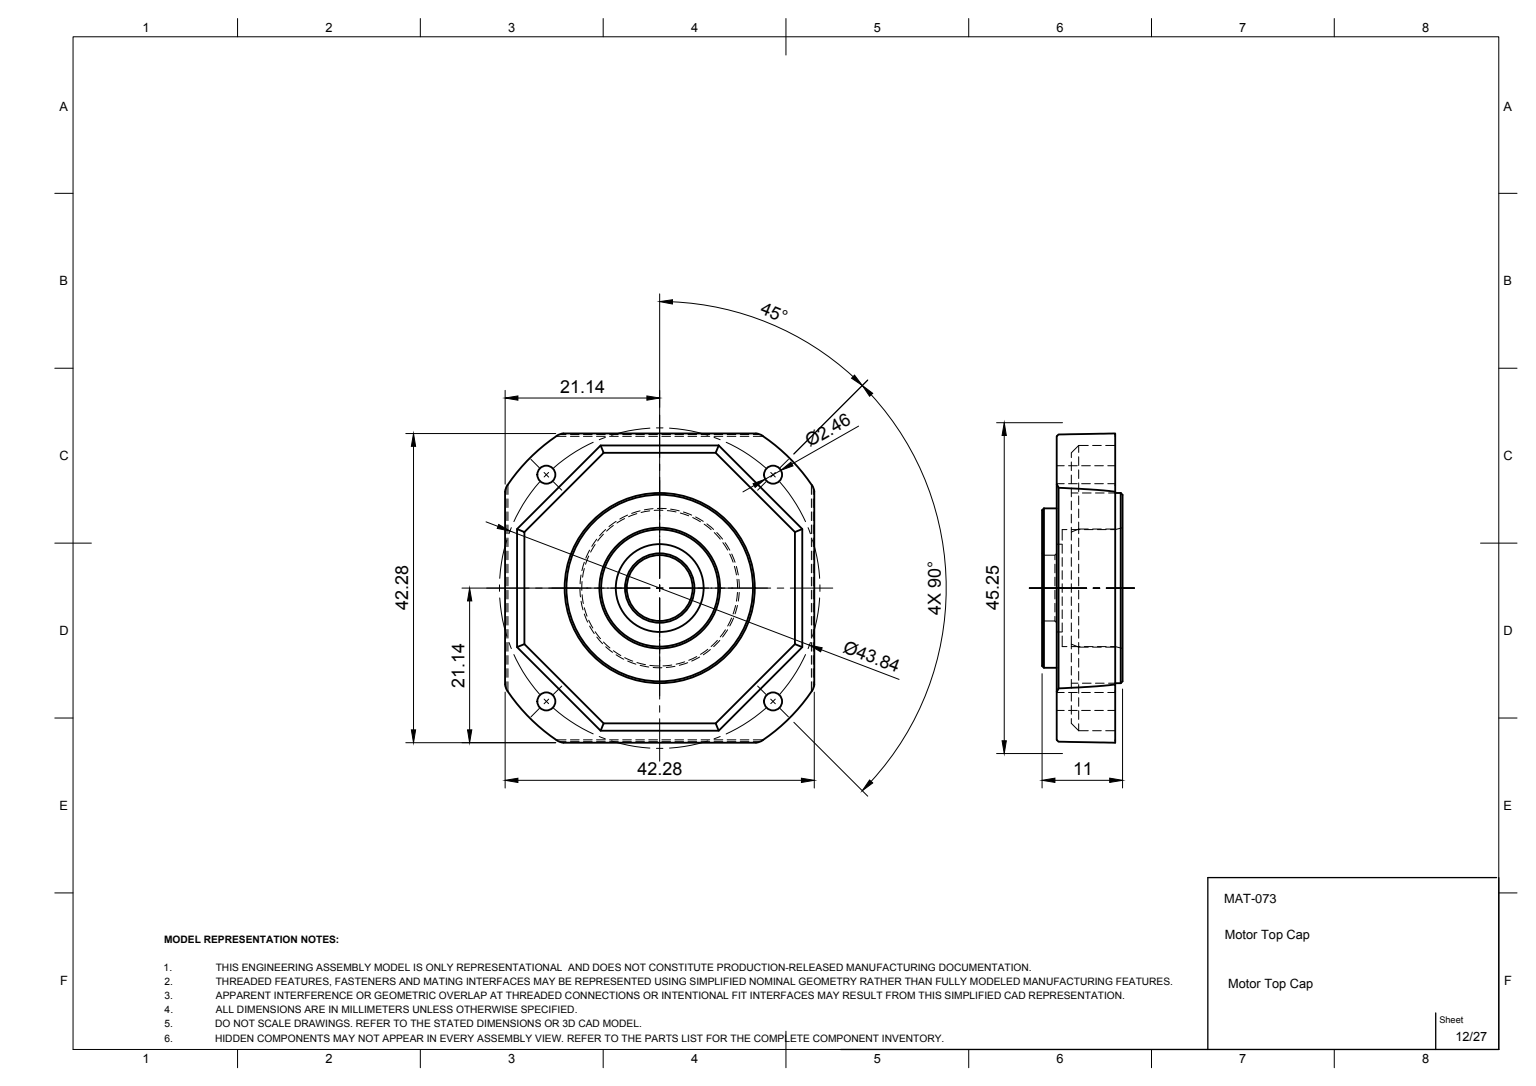
ISO-10303-21;
HEADER;
/* Generated by software containing ST-Developer
 * from STEP Tools, Inc. (www.steptools.com) 
 */

FILE_DESCRIPTION(
/* description */ ('CAx-IF Rec.Pracs.---Representation and Presentation of Product Manufa
cturing Information (PMI)---4.0---2014-10-13'),
/* implementation_level */ '2;1');

FILE_NAME(
/* name */ 'Motor Top Cap.step',
/* time_stamp */ '2026-10-24T18:52:33-07:00',
/* author */ (''),
/* organization */ (''),
/* preprocessor_version */ 'ST-DEVELOPER v20.2',
/* originating_system */ 'Autodesk Translation Framework v15.17.0.0',
/* authorisation */ '');

FILE_SCHEMA (('AP242_MANAGED_MODEL_BASED_3D_ENGINEERING_MIM_LF { 1 0 10303 442 2 1 4 }'));
ENDSEC;

DATA;
#10=MECHANICAL_DESIGN_GEOMETRIC_PRESENTATION_REPRESENTATION('',(#425),#34876);
#180=CONICAL_SURFACE('',#21050,0.010775,0.785398163397447);
#181=CONICAL_SURFACE('',#21057,0.004625,0.785398163397445);
#182=CONICAL_SURFACE('',#21062,0.004625,0.785398163397443);
#183=CONICAL_SURFACE('',#21066,0.012875,0.785398163397446);
#184=CONICAL_SURFACE('',#21072,0.008125,0.244978663126864);
#324=ELLIPSE('',#20968,0.00280406412975229,0.00200000000000295);
#325=ELLIPSE('',#20969,0.114597376997271,0.00200000000000295);
#326=ELLIPSE('',#20972,0.0352260556300016,0.0251250000000291);
#327=ELLIPSE('',#20974,0.0352260556300019,0.0251250000000291);
#328=ELLIPSE('',#20977,0.00280406412976774,0.00200000000001397);
#329=ELLIPSE('',#20978,0.114597376997902,0.00200000000001397);
#330=ELLIPSE('',#20981,0.0352260556299788,0.0251250000000126);
#331=ELLIPSE('',#20983,0.0352260556299788,0.0251250000000126);
#332=ELLIPSE('',#20986,0.00280406412974482,0.00199999999999762);
#333=ELLIPSE('',#20987,0.114597376996966,0.00199999999999762);
#334=ELLIPSE('',#20990,0.0352260556299805,0.0251250000000138);
#335=ELLIPSE('',#20992,0.0352260556299805,0.0251250000000138);
#336=ELLIPSE('',#20995,0.00280406412972858,0.00199999999998605);
#337=ELLIPSE('',#20996,0.114597376996303,0.00199999999998605);
#338=ELLIPSE('',#20999,0.0352260556299806,0.0251250000000138);
#339=ELLIPSE('',#21001,0.0352260556299803,0.0251250000000138);
#340=ELLIPSE('',#21004,0.114597376996528,0.00199999999998998);
#341=ELLIPSE('',#21005,0.00280406412973409,0.00199999999998998);
#342=ELLIPSE('',#21008,0.114597376996513,0.00199999999998973);
#343=ELLIPSE('',#21009,0.00280406412973375,0.00199999999998973);
#344=ELLIPSE('',#21012,0.114597376996527,0.00199999999998997);
#345=ELLIPSE('',#21013,0.00280406412973409,0.00199999999998997);
#346=ELLIPSE('',#21016,0.114597376997844,0.00200000000001296);
#347=ELLIPSE('',#21017,0.00280406412976633,0.00200000000001296);
#359=SHAPE_REPRESENTATION_RELATIONSHIP('SRR','None',#34996,#392);
#392=ADVANCED_BREP_SHAPE_REPRESENTATION('',(#458),#34854);
#425=STYLED_ITEM('',(#35162),#458);
#458=MANIFOLD_SOLID_BREP('Motor Top Cap',#19565);
#519=FACE_BOUND('',#6354,.T.);
#520=FACE_BOUND('',#6355,.T.);
#521=FACE_BOUND('',#6356,.T.);
#522=FACE_BOUND('',#6357,.T.);
#523=FACE_BOUND('',#6358,.T.);
#524=FACE_BOUND('',#6361,.T.);
#525=FACE_BOUND('',#6362,.T.);
#526=FACE_BOUND('',#6363,.T.);
#527=FACE_BOUND('',#6364,.T.);
#528=FACE_BOUND('',#6365,.T.);
#529=FACE_BOUND('',#6379,.T.);
#530=FACE_BOUND('',#6383,.T.);
#531=FACE_BOUND('',#6389,.T.);
#532=FACE_BOUND('',#6392,.T.);
#533=FACE_BOUND('',#6402,.T.);
#816=PLANE('',#21018);
#817=PLANE('',#21019);
#818=PLANE('',#21020);
#819=PLANE('',#21021);
#820=PLANE('',#21022);
#821=PLANE('',#21023);
#822=PLANE('',#21028);
#823=PLANE('',#21029);
#824=PLANE('',#21035);
#825=PLANE('',#21036);
#826=PLANE('',#21037);
#827=PLANE('',#21038);
#828=PLANE('',#21039);
#829=PLANE('',#21040);
#830=PLANE('',#21041);
#831=PLANE('',#21042);
#832=PLANE('',#21043);
#833=PLANE('',#21044);
#834=PLANE('',#21045);
#835=PLANE('',#21046);
#836=PLANE('',#21047);
#837=PLANE('',#21049);
#838=PLANE('',#21054);
#839=PLANE('',#21064);
#840=PLANE('',#21069);
#841=PLANE('',#21083);
#842=PLANE('',#21084);
#843=PLANE('',#21085);
#844=PLANE('',#21086);
#845=PLANE('',#21087);
#846=PLANE('',#21088);
#1767=LINE('',#31314,#3366);
#1768=LINE('',#31322,#3367);
#1769=LINE('',#31333,#3368);
#1770=LINE('',#31341,#3369);
#1771=LINE('',#31352,#3370);
#1772=LINE('',#31360,#3371);
#1773=LINE('',#31371,#3372);
#1774=LINE('',#31379,#3373);
#1775=LINE('',#31410,#3374);
#1776=LINE('',#31411,#3375);
#1777=LINE('',#31413,#3376);
#1778=LINE('',#31415,#3377);
#1779=LINE('',#31416,#3378);
#1780=LINE('',#31418,#3379);
#1781=LINE('',#31420,#3380);
#1782=LINE('',#31421,#3381);
#1783=LINE('',#31423,#3382);
#1784=LINE('',#31426,#3383);
#1785=LINE('',#31428,#3384);
#1786=LINE('',#31430,#3385);
#1787=LINE('',#31432,#3386);
#1788=LINE('',#31434,#3387);
#1789=LINE('',#31436,#3388);
#1790=LINE('',#31438,#3389);
#1791=LINE('',#31439,#3390);
#1792=LINE('',#31449,#3391);
#1793=LINE('',#31451,#3392);
#1794=LINE('',#31465,#3393);
#1795=LINE('',#31467,#3394);
#1796=LINE('',#31469,#3395);
#1797=LINE('',#31470,#3396);
#1798=LINE('',#31473,#3397);
#1799=LINE('',#31475,#3398);
#1800=LINE('',#31476,#3399);
#1801=LINE('',#31479,#3400);
#1802=LINE('',#31481,#3401);
#1803=LINE('',#31482,#3402);
#1804=LINE('',#31485,#3403);
#1805=LINE('',#31487,#3404);
#1806=LINE('',#31488,#3405);
#1807=LINE('',#31491,#3406);
#1808=LINE('',#31493,#3407);
#1809=LINE('',#31494,#3408);
#1810=LINE('',#31497,#3409);
#1811=LINE('',#31499,#3410);
#1812=LINE('',#31500,#3411);
#1813=LINE('',#31503,#3412);
#1814=LINE('',#31505,#3413);
#1815=LINE('',#31506,#3414);
#1816=LINE('',#31508,#3415);
#1817=LINE('',#31509,#3416);
#1818=LINE('',#31511,#3417);
#1819=LINE('',#31512,#3418);
#1820=LINE('',#31514,#3419);
#1821=LINE('',#31516,#3420);
#1822=LINE('',#31518,#3421);
#1823=LINE('',#31523,#3422);
#1824=LINE('',#31529,#3423);
#1825=LINE('',#31536,#3424);
#1826=LINE('',#31541,#3425);
#1827=LINE('',#31546,#3426);
#1828=LINE('',#31549,#3427);
#1829=LINE('',#31558,#3428);
#1830=LINE('',#31564,#3429);
#1831=LINE('',#31569,#3430);
#1832=LINE('',#31573,#3431);
#1833=LINE('',#31576,#3432);
#1834=LINE('',#31578,#3433);
#1835=LINE('',#31580,#3434);
#1836=LINE('',#31582,#3435);
#1837=LINE('',#31586,#3436);
#1838=LINE('',#31589,#3437);
#1839=LINE('',#31591,#3438);
#1840=LINE('',#31593,#3439);
#3366=VECTOR('',#24976,0.01);
#3367=VECTOR('',#24985,0.01);
#3368=VECTOR('',#24996,0.01);
#3369=VECTOR('',#25005,0.01);
#3370=VECTOR('',#25016,0.01);
#3371=VECTOR('',#25025,0.01);
#3372=VECTOR('',#25036,0.01);
#3373=VECTOR('',#25045,0.01);
#3374=VECTOR('',#25086,1.);
#3375=VECTOR('',#25087,1.);
#3376=VECTOR('',#25090,1.);
#3377=VECTOR('',#25093,1.);
#3378=VECTOR('',#25094,1.);
#3379=VECTOR('',#25097,1.);
#3380=VECTOR('',#25100,1.);
#3381=VECTOR('',#25101,1.);
#3382=VECTOR('',#25104,1.);
#3383=VECTOR('',#25105,1.);
#3384=VECTOR('',#25106,1.);
#3385=VECTOR('',#25107,1.);
#3386=VECTOR('',#25108,1.);
#3387=VECTOR('',#25109,1.);
#3388=VECTOR('',#25110,1.);
#3389=VECTOR('',#25111,1.);
#3390=VECTOR('',#25112,1.);
#3391=VECTOR('',#25123,1.);
#3392=VECTOR('',#25126,1.);
#3393=VECTOR('',#25139,1.);
#3394=VECTOR('',#25140,1.);
#3395=VECTOR('',#25141,1.);
#3396=VECTOR('',#25142,1.);
#3397=VECTOR('',#25145,1.);
#3398=VECTOR('',#25146,1.);
#3399=VECTOR('',#25147,1.);
#3400=VECTOR('',#25150,1.);
#3401=VECTOR('',#25151,1.);
#3402=VECTOR('',#25152,1.);
#3403=VECTOR('',#25155,1.);
#3404=VECTOR('',#25156,1.);
#3405=VECTOR('',#25157,1.);
#3406=VECTOR('',#25160,1.);
#3407=VECTOR('',#25161,1.);
#3408=VECTOR('',#25162,1.);
#3409=VECTOR('',#25165,1.);
#3410=VECTOR('',#25166,1.);
#3411=VECTOR('',#25167,1.);
#3412=VECTOR('',#25170,1.);
#3413=VECTOR('',#25171,1.);
#3414=VECTOR('',#25172,1.);
#3415=VECTOR('',#25175,1.);
#3416=VECTOR('',#25176,1.);
#3417=VECTOR('',#25179,1.);
#3418=VECTOR('',#25180,1.);
#3419=VECTOR('',#25183,1.);
#3420=VECTOR('',#25186,1.);
#3421=VECTOR('',#25189,1.);
#3422=VECTOR('',#25196,1.);
#3423=VECTOR('',#25201,0.010775);
#3424=VECTOR('',#25212,0.0109);
#3425=VECTOR('',#25217,0.004625);
#3426=VECTOR('',#25224,0.0045);
#3427=VECTOR('',#25227,0.004625);
#3428=VECTOR('',#25238,0.012875);
#3429=VECTOR('',#25247,0.013);
#3430=VECTOR('',#25252,0.008125);
#3431=VECTOR('',#25257,0.008);
#3432=VECTOR('',#25262,0.0012295);
#3433=VECTOR('',#25265,0.0012295);
#3434=VECTOR('',#25268,0.0012295);
#3435=VECTOR('',#25271,0.0012295);
#3436=VECTOR('',#25276,0.006);
#3437=VECTOR('',#25281,1.);
#3438=VECTOR('',#25284,1.);
#3439=VECTOR('',#25287,1.);
#4504=CYLINDRICAL_SURFACE('',#20966,0.00200000000000295);
#4505=CYLINDRICAL_SURFACE('',#20970,0.0251250000000291);
#4506=CYLINDRICAL_SURFACE('',#20975,0.00200000000001397);
#4507=CYLINDRICAL_SURFACE('',#20979,0.0251250000000126);
#4508=CYLINDRICAL_SURFACE('',#20984,0.00199999999999762);
#4509=CYLINDRICAL_SURFACE('',#20988,0.0251250000000138);
#4510=CYLINDRICAL_SURFACE('',#20993,0.00199999999998605);
#4511=CYLINDRICAL_SURFACE('',#20997,0.0251250000000138);
#4512=CYLINDRICAL_SURFACE('',#21002,0.00199999999998998);
#4513=CYLINDRICAL_SURFACE('',#21006,0.00199999999998973);
#4514=CYLINDRICAL_SURFACE('',#21010,0.00199999999998997);
#4515=CYLINDRICAL_SURFACE('',#21014,0.00200000000001296);
#4516=CYLINDRICAL_SURFACE('',#21056,0.0109);
#4517=CYLINDRICAL_SURFACE('',#21060,0.0045);
#4518=CYLINDRICAL_SURFACE('',#21071,0.013);
#4519=CYLINDRICAL_SURFACE('',#21075,0.008);
#4520=CYLINDRICAL_SURFACE('',#21077,0.0012295);
#4521=CYLINDRICAL_SURFACE('',#21078,0.0012295);
#4522=CYLINDRICAL_SURFACE('',#21079,0.0012295);
#4523=CYLINDRICAL_SURFACE('',#21080,0.0012295);
#4524=CYLINDRICAL_SURFACE('',#21081,0.006);
#5252=FACE_OUTER_BOUND('',#6336,.T.);
#5253=FACE_OUTER_BOUND('',#6337,.T.);
#5254=FACE_OUTER_BOUND('',#6338,.T.);
#5255=FACE_OUTER_BOUND('',#6339,.T.);
#5256=FACE_OUTER_BOUND('',#6340,.T.);
#5257=FACE_OUTER_BOUND('',#6341,.T.);
#5258=FACE_OUTER_BOUND('',#6342,.T.);
#5259=FACE_OUTER_BOUND('',#6343,.T.);
#5260=FACE_OUTER_BOUND('',#6344,.T.);
#5261=FACE_OUTER_BOUND('',#6345,.T.);
#5262=FACE_OUTER_BOUND('',#6346,.T.);
#5263=FACE_OUTER_BOUND('',#6347,.T.);
#5264=FACE_OUTER_BOUND('',#6348,.T.);
#5265=FACE_OUTER_BOUND('',#6349,.T.);
#5266=FACE_OUTER_BOUND('',#6350,.T.);
#5267=FACE_OUTER_BOUND('',#6351,.T.);
#5268=FACE_OUTER_BOUND('',#6352,.T.);
#5269=FACE_OUTER_BOUND('',#6353,.T.);
#5270=FACE_OUTER_BOUND('',#6359,.T.);
#5271=FACE_OUTER_BOUND('',#6360,.T.);
#5272=FACE_OUTER_BOUND('',#6366,.T.);
#5273=FACE_OUTER_BOUND('',#6367,.T.);
#5274=FACE_OUTER_BOUND('',#6368,.T.);
#5275=FACE_OUTER_BOUND('',#6369,.T.);
#5276=FACE_OUTER_BOUND('',#6370,.T.);
#5277=FACE_OUTER_BOUND('',#6371,.T.);
#5278=FACE_OUTER_BOUND('',#6372,.T.);
#5279=FACE_OUTER_BOUND('',#6373,.T.);
#5280=FACE_OUTER_BOUND('',#6374,.T.);
#5281=FACE_OUTER_BOUND('',#6375,.T.);
#5282=FACE_OUTER_BOUND('',#6376,.T.);
#5283=FACE_OUTER_BOUND('',#6377,.T.);
#5284=FACE_OUTER_BOUND('',#6378,.T.);
#5285=FACE_OUTER_BOUND('',#6380,.T.);
#5286=FACE_OUTER_BOUND('',#6381,.T.);
#5287=FACE_OUTER_BOUND('',#6382,.T.);
#5288=FACE_OUTER_BOUND('',#6384,.T.);
#5289=FACE_OUTER_BOUND('',#6385,.T.);
#5290=FACE_OUTER_BOUND('',#6386,.T.);
#5291=FACE_OUTER_BOUND('',#6387,.T.);
#5292=FACE_OUTER_BOUND('',#6388,.T.);
#5293=FACE_OUTER_BOUND('',#6390,.T.);
#5294=FACE_OUTER_BOUND('',#6391,.T.);
#5295=FACE_OUTER_BOUND('',#6393,.T.);
#5296=FACE_OUTER_BOUND('',#6394,.T.);
#5297=FACE_OUTER_BOUND('',#6395,.T.);
#5298=FACE_OUTER_BOUND('',#6396,.T.);
#5299=FACE_OUTER_BOUND('',#6397,.T.);
#5300=FACE_OUTER_BOUND('',#6398,.T.);
#5301=FACE_OUTER_BOUND('',#6399,.T.);
#5302=FACE_OUTER_BOUND('',#6400,.T.);
#5303=FACE_OUTER_BOUND('',#6401,.T.);
#5304=FACE_OUTER_BOUND('',#6403,.T.);
#5305=FACE_OUTER_BOUND('',#6404,.T.);
#5306=FACE_OUTER_BOUND('',#6405,.T.);
#5307=FACE_OUTER_BOUND('',#6406,.T.);
#5308=FACE_OUTER_BOUND('',#6407,.T.);
#6336=EDGE_LOOP('',(#15300,#15301,#15302,#15303));
#6337=EDGE_LOOP('',(#15304,#15305,#15306,#15307,#15308,#15309));
#6338=EDGE_LOOP('',(#15310,#15311,#15312,#15313));
#6339=EDGE_LOOP('',(#15314,#15315,#15316,#15317,#15318,#15319));
#6340=EDGE_LOOP('',(#15320,#15321,#15322,#15323));
#6341=EDGE_LOOP('',(#15324,#15325,#15326,#15327,#15328,#15329));
#6342=EDGE_LOOP('',(#15330,#15331,#15332,#15333));
#6343=EDGE_LOOP('',(#15334,#15335,#15336,#15337,#15338,#15339));
#6344=EDGE_LOOP('',(#15340,#15341,#15342,#15343));
#6345=EDGE_LOOP('',(#15344,#15345,#15346,#15347));
#6346=EDGE_LOOP('',(#15348,#15349,#15350,#15351));
#6347=EDGE_LOOP('',(#15352,#15353,#15354,#15355));
#6348=EDGE_LOOP('',(#15356,#15357,#15358,#15359));
#6349=EDGE_LOOP('',(#15360,#15361,#15362,#15363,#15364,#15365));
#6350=EDGE_LOOP('',(#15366,#15367,#15368,#15369));
#6351=EDGE_LOOP('',(#15370,#15371,#15372,#15373,#15374,#15375));
#6352=EDGE_LOOP('',(#15376,#15377,#15378,#15379));
#6353=EDGE_LOOP('',(#15380,#15381,#15382,#15383,#15384,#15385,#15386,#15387,
#15388,#15389,#15390,#15391,#15392,#15393,#15394,#15395));
#6354=EDGE_LOOP('',(#15396,#15397,#15398,#15399,#15400,#15401,#15402,#15403));
#6355=EDGE_LOOP('',(#15404));
#6356=EDGE_LOOP('',(#15405));
#6357=EDGE_LOOP('',(#15406));
#6358=EDGE_LOOP('',(#15407));
#6359=EDGE_LOOP('',(#15408,#15409,#15410,#15411,#15412,#15413));
#6360=EDGE_LOOP('',(#15414,#15415,#15416,#15417,#15418,#15419,#15420,#15421));
#6361=EDGE_LOOP('',(#15422));
#6362=EDGE_LOOP('',(#15423));
#6363=EDGE_LOOP('',(#15424));
#6364=EDGE_LOOP('',(#15425));
#6365=EDGE_LOOP('',(#15426));
#6366=EDGE_LOOP('',(#15427,#15428,#15429,#15430));
#6367=EDGE_LOOP('',(#15431,#15432,#15433,#15434));
#6368=EDGE_LOOP('',(#15435,#15436,#15437,#15438));
#6369=EDGE_LOOP('',(#15439,#15440,#15441,#15442));
#6370=EDGE_LOOP('',(#15443,#15444,#15445,#15446));
#6371=EDGE_LOOP('',(#15447,#15448,#15449,#15450));
#6372=EDGE_LOOP('',(#15451,#15452,#15453,#15454));
#6373=EDGE_LOOP('',(#15455,#15456,#15457,#15458));
#6374=EDGE_LOOP('',(#15459,#15460,#15461,#15462));
#6375=EDGE_LOOP('',(#15463,#15464,#15465,#15466));
#6376=EDGE_LOOP('',(#15467,#15468,#15469,#15470));
#6377=EDGE_LOOP('',(#15471,#15472,#15473,#15474));
#6378=EDGE_LOOP('',(#15475,#15476,#15477,#15478,#15479,#15480,#15481,#15482));
#6379=EDGE_LOOP('',(#15483));
#6380=EDGE_LOOP('',(#15484,#15485,#15486,#15487,#15488,#15489));
#6381=EDGE_LOOP('',(#15490,#15491,#15492,#15493,#15494));
#6382=EDGE_LOOP('',(#15495));
#6383=EDGE_LOOP('',(#15496));
#6384=EDGE_LOOP('',(#15497,#15498,#15499,#15500,#15501));
#6385=EDGE_LOOP('',(#15502,#15503,#15504,#15505,#15506));
#6386=EDGE_LOOP('',(#15507,#15508,#15509,#15510,#15511));
#6387=EDGE_LOOP('',(#15512,#15513,#15514,#15515));
#6388=EDGE_LOOP('',(#15516));
#6389=EDGE_LOOP('',(#15517));
#6390=EDGE_LOOP('',(#15518,#15519,#15520,#15521));
#6391=EDGE_LOOP('',(#15522));
#6392=EDGE_LOOP('',(#15523));
#6393=EDGE_LOOP('',(#15524,#15525,#15526,#15527));
#6394=EDGE_LOOP('',(#15528,#15529,#15530,#15531,#15532));
#6395=EDGE_LOOP('',(#15533,#15534,#15535,#15536,#15537));
#6396=EDGE_LOOP('',(#15538,#15539,#15540,#15541));
#6397=EDGE_LOOP('',(#15542,#15543,#15544,#15545));
#6398=EDGE_LOOP('',(#15546,#15547,#15548,#15549));
#6399=EDGE_LOOP('',(#15550,#15551,#15552,#15553));
#6400=EDGE_LOOP('',(#15554,#15555,#15556,#15557));
#6401=EDGE_LOOP('',(#15558));
#6402=EDGE_LOOP('',(#15559));
#6403=EDGE_LOOP('',(#15560,#15561,#15562,#15563));
#6404=EDGE_LOOP('',(#15564,#15565,#15566,#15567));
#6405=EDGE_LOOP('',(#15568,#15569,#15570,#15571));
#6406=EDGE_LOOP('',(#15572,#15573,#15574,#15575));
#6407=EDGE_LOOP('',(#15576,#15577,#15578,#15579));
#7448=CIRCLE('',#20967,0.00200000000000295);
#7449=CIRCLE('',#20971,0.0251250000000291);
#7450=CIRCLE('',#20973,0.0251250000000291);
#7451=CIRCLE('',#20976,0.00200000000001397);
#7452=CIRCLE('',#20980,0.0251250000000126);
#7453=CIRCLE('',#20982,0.0251250000000126);
#7454=CIRCLE('',#20985,0.00199999999999762);
#7455=CIRCLE('',#20989,0.0251250000000138);
#7456=CIRCLE('',#20991,0.0251250000000138);
#7457=CIRCLE('',#20994,0.00199999999998605);
#7458=CIRCLE('',#20998,0.0251250000000138);
#7459=CIRCLE('',#21000,0.0251250000000138);
#7460=CIRCLE('',#21003,0.00199999999998998);
#7461=CIRCLE('',#21007,0.00199999999998973);
#7462=CIRCLE('',#21011,0.00199999999998997);
#7463=CIRCLE('',#21015,0.00200000000001296);
#7464=CIRCLE('',#21024,0.00122950000001);
#7465=CIRCLE('',#21025,0.00122950000001);
#7466=CIRCLE('',#21026,0.00122950000001);
#7467=CIRCLE('',#21027,0.00122950000001);
#7468=CIRCLE('',#21030,0.00122950000001);
#7469=CIRCLE('',#21031,0.00122950000001);
#7470=CIRCLE('',#21032,0.00122950000001);
#7471=CIRCLE('',#21033,0.00122950000001);
#7472=CIRCLE('',#21034,0.01090000000001);
#7473=CIRCLE('',#21048,0.01300000000001);
#7474=CIRCLE('',#21051,0.01090000000001);
#7475=CIRCLE('',#21052,0.01065000000001);
#7476=CIRCLE('',#21053,0.01090000000001);
#7477=CIRCLE('',#21055,0.00475000000001);
#7478=CIRCLE('',#21058,0.00450000000001);
#7479=CIRCLE('',#21059,0.00450000000001);
#7480=CIRCLE('',#21061,0.00450000000001);
#7481=CIRCLE('',#21063,0.00475000000001);
#7482=CIRCLE('',#21065,0.00600000000001);
#7483=CIRCLE('',#21067,0.01300000000001);
#7484=CIRCLE('',#21068,0.01275000000001);
#7485=CIRCLE('',#21070,0.00825000000001);
#7486=CIRCLE('',#21073,0.00800000000001);
#7487=CIRCLE('',#21074,0.00800000000001);
#7488=CIRCLE('',#21076,0.00800000000001);
#7489=CIRCLE('',#21082,0.00600000000001);
#8900=VERTEX_POINT('',#31310);
#8901=VERTEX_POINT('',#31311);
#8902=VERTEX_POINT('',#31313);
#8903=VERTEX_POINT('',#31315);
#8904=VERTEX_POINT('',#31319);
#8905=VERTEX_POINT('',#31321);
#8906=VERTEX_POINT('',#31323);
#8907=VERTEX_POINT('',#31325);
#8908=VERTEX_POINT('',#31329);
#8909=VERTEX_POINT('',#31330);
#8910=VERTEX_POINT('',#31332);
#8911=VERTEX_POINT('',#31334);
#8912=VERTEX_POINT('',#31338);
#8913=VERTEX_POINT('',#31340);
#8914=VERTEX_POINT('',#31342);
#8915=VERTEX_POINT('',#31344);
#8916=VERTEX_POINT('',#31348);
#8917=VERTEX_POINT('',#31349);
#8918=VERTEX_POINT('',#31351);
#8919=VERTEX_POINT('',#31353);
#8920=VERTEX_POINT('',#31357);
#8921=VERTEX_POINT('',#31359);
#8922=VERTEX_POINT('',#31361);
#8923=VERTEX_POINT('',#31363);
#8924=VERTEX_POINT('',#31367);
#8925=VERTEX_POINT('',#31368);
#8926=VERTEX_POINT('',#31370);
#8927=VERTEX_POINT('',#31372);
#8928=VERTEX_POINT('',#31376);
#8929=VERTEX_POINT('',#31378);
#8930=VERTEX_POINT('',#31380);
#8931=VERTEX_POINT('',#31382);
#8932=VERTEX_POINT('',#31386);
#8933=VERTEX_POINT('',#31388);
#8934=VERTEX_POINT('',#31392);
#8935=VERTEX_POINT('',#31394);
#8936=VERTEX_POINT('',#31398);
#8937=VERTEX_POINT('',#31400);
#8938=VERTEX_POINT('',#31404);
#8939=VERTEX_POINT('',#31406);
#8940=VERTEX_POINT('',#31424);
#8941=VERTEX_POINT('',#31425);
#8942=VERTEX_POINT('',#31427);
#8943=VERTEX_POINT('',#31429);
#8944=VERTEX_POINT('',#31431);
#8945=VERTEX_POINT('',#31433);
#8946=VERTEX_POINT('',#31435);
#8947=VERTEX_POINT('',#31437);
#8948=VERTEX_POINT('',#31440);
#8949=VERTEX_POINT('',#31442);
#8950=VERTEX_POINT('',#31444);
#8951=VERTEX_POINT('',#31446);
#8952=VERTEX_POINT('',#31452);
#8953=VERTEX_POINT('',#31454);
#8954=VERTEX_POINT('',#31456);
#8955=VERTEX_POINT('',#31458);
#8956=VERTEX_POINT('',#31460);
#8957=VERTEX_POINT('',#31463);
#8958=VERTEX_POINT('',#31464);
#8959=VERTEX_POINT('',#31466);
#8960=VERTEX_POINT('',#31468);
#8961=VERTEX_POINT('',#31472);
#8962=VERTEX_POINT('',#31474);
#8963=VERTEX_POINT('',#31478);
#8964=VERTEX_POINT('',#31480);
#8965=VERTEX_POINT('',#31484);
#8966=VERTEX_POINT('',#31486);
#8967=VERTEX_POINT('',#31490);
#8968=VERTEX_POINT('',#31492);
#8969=VERTEX_POINT('',#31496);
#8970=VERTEX_POINT('',#31498);
#8971=VERTEX_POINT('',#31502);
#8972=VERTEX_POINT('',#31504);
#8973=VERTEX_POINT('',#31520);
#8974=VERTEX_POINT('',#31525);
#8975=VERTEX_POINT('',#31526);
#8976=VERTEX_POINT('',#31528);
#8977=VERTEX_POINT('',#31533);
#8978=VERTEX_POINT('',#31538);
#8979=VERTEX_POINT('',#31539);
#8980=VERTEX_POINT('',#31544);
#8981=VERTEX_POINT('',#31548);
#8982=VERTEX_POINT('',#31552);
#8983=VERTEX_POINT('',#31555);
#8984=VERTEX_POINT('',#31557);
#8985=VERTEX_POINT('',#31561);
#8986=VERTEX_POINT('',#31566);
#8987=VERTEX_POINT('',#31567);
#8988=VERTEX_POINT('',#31572);
#8989=VERTEX_POINT('',#31584);
#11208=EDGE_CURVE('',#8900,#8901,#7448,.T.);
#11209=EDGE_CURVE('',#8902,#8900,#1767,.T.);
#11210=EDGE_CURVE('',#8903,#8902,#324,.T.);
#11211=EDGE_CURVE('',#8901,#8903,#325,.T.);
#11212=EDGE_CURVE('',#8904,#8900,#7449,.T.);
#11213=EDGE_CURVE('',#8905,#8904,#1768,.T.);
#11214=EDGE_CURVE('',#8906,#8905,#326,.T.);
#11215=EDGE_CURVE('',#8907,#8906,#7450,.T.);
#11216=EDGE_CURVE('',#8902,#8907,#327,.T.);
#11217=EDGE_CURVE('',#8908,#8909,#7451,.T.);
#11218=EDGE_CURVE('',#8910,#8908,#1769,.T.);
#11219=EDGE_CURVE('',#8911,#8910,#328,.T.);
#11220=EDGE_CURVE('',#8909,#8911,#329,.T.);
#11221=EDGE_CURVE('',#8912,#8908,#7452,.T.);
#11222=EDGE_CURVE('',#8913,#8912,#1770,.T.);
#11223=EDGE_CURVE('',#8914,#8913,#330,.T.);
#11224=EDGE_CURVE('',#8915,#8914,#7453,.T.);
#11225=EDGE_CURVE('',#8910,#8915,#331,.T.);
#11226=EDGE_CURVE('',#8916,#8917,#7454,.T.);
#11227=EDGE_CURVE('',#8918,#8916,#1771,.T.);
#11228=EDGE_CURVE('',#8919,#8918,#332,.T.);
#11229=EDGE_CURVE('',#8917,#8919,#333,.T.);
#11230=EDGE_CURVE('',#8920,#8916,#7455,.T.);
#11231=EDGE_CURVE('',#8921,#8920,#1772,.T.);
#11232=EDGE_CURVE('',#8922,#8921,#334,.T.);
#11233=EDGE_CURVE('',#8923,#8922,#7456,.T.);
#11234=EDGE_CURVE('',#8918,#8923,#335,.T.);
#11235=EDGE_CURVE('',#8924,#8925,#7457,.T.);
#11236=EDGE_CURVE('',#8926,#8924,#1773,.T.);
#11237=EDGE_CURVE('',#8927,#8926,#336,.T.);
#11238=EDGE_CURVE('',#8925,#8927,#337,.T.);
#11239=EDGE_CURVE('',#8928,#8924,#7458,.T.);
#11240=EDGE_CURVE('',#8929,#8928,#1774,.T.);
#11241=EDGE_CURVE('',#8930,#8929,#338,.T.);
#11242=EDGE_CURVE('',#8931,#8930,#7459,.T.);
#11243=EDGE_CURVE('',#8926,#8931,#339,.T.);
#11244=EDGE_CURVE('',#8932,#8904,#7460,.T.);
#11245=EDGE_CURVE('',#8933,#8932,#340,.T.);
#11246=EDGE_CURVE('',#8905,#8933,#341,.T.);
#11247=EDGE_CURVE('',#8934,#8912,#7461,.T.);
#11248=EDGE_CURVE('',#8935,#8934,#342,.T.);
#11249=EDGE_CURVE('',#8913,#8935,#343,.T.);
#11250=EDGE_CURVE('',#8936,#8920,#7462,.T.);
#11251=EDGE_CURVE('',#8937,#8936,#344,.T.);
#11252=EDGE_CURVE('',#8921,#8937,#345,.T.);
#11253=EDGE_CURVE('',#8938,#8928,#7463,.T.);
#11254=EDGE_CURVE('',#8939,#8938,#346,.T.);
#11255=EDGE_CURVE('',#8929,#8939,#347,.T.);
#11256=EDGE_CURVE('',#8935,#8903,#1775,.T.);
#11257=EDGE_CURVE('',#8934,#8901,#1776,.T.);
#11258=EDGE_CURVE('',#8907,#8914,#1777,.T.);
#11259=EDGE_CURVE('',#8937,#8911,#1778,.T.);
#11260=EDGE_CURVE('',#8936,#8909,#1779,.T.);
#11261=EDGE_CURVE('',#8915,#8922,#1780,.T.);
#11262=EDGE_CURVE('',#8939,#8919,#1781,.T.);
#11263=EDGE_CURVE('',#8938,#8917,#1782,.T.);
#11264=EDGE_CURVE('',#8932,#8925,#1783,.T.);
#11265=EDGE_CURVE('',#8940,#8941,#1784,.T.);
#11266=EDGE_CURVE('',#8941,#8942,#1785,.T.);
#11267=EDGE_CURVE('',#8942,#8943,#1786,.T.);
#11268=EDGE_CURVE('',#8943,#8944,#1787,.T.);
#11269=EDGE_CURVE('',#8944,#8945,#1788,.T.);
#11270=EDGE_CURVE('',#8945,#8946,#1789,.T.);
#11271=EDGE_CURVE('',#8946,#8947,#1790,.T.);
#11272=EDGE_CURVE('',#8947,#8940,#1791,.T.);
#11273=EDGE_CURVE('',#8948,#8948,#7464,.T.);
#11274=EDGE_CURVE('',#8949,#8949,#7465,.T.);
#11275=EDGE_CURVE('',#8950,#8950,#7466,.T.);
#11276=EDGE_CURVE('',#8951,#8951,#7467,.T.);
#11277=EDGE_CURVE('',#8923,#8930,#1792,.T.);
#11278=EDGE_CURVE('',#8931,#8906,#1793,.T.);
#11279=EDGE_CURVE('',#8952,#8952,#7468,.T.);
#11280=EDGE_CURVE('',#8953,#8953,#7469,.T.);
#11281=EDGE_CURVE('',#8954,#8954,#7470,.T.);
#11282=EDGE_CURVE('',#8955,#8955,#7471,.T.);
#11283=EDGE_CURVE('',#8956,#8956,#7472,.T.);
#11284=EDGE_CURVE('',#8957,#8958,#1794,.T.);
#11285=EDGE_CURVE('',#8958,#8959,#1795,.T.);
#11286=EDGE_CURVE('',#8959,#8960,#1796,.T.);
#11287=EDGE_CURVE('',#8957,#8960,#1797,.T.);
#11288=EDGE_CURVE('',#8958,#8961,#1798,.T.);
#11289=EDGE_CURVE('',#8961,#8962,#1799,.T.);
#11290=EDGE_CURVE('',#8962,#8959,#1800,.T.);
#11291=EDGE_CURVE('',#8961,#8963,#1801,.T.);
#11292=EDGE_CURVE('',#8963,#8964,#1802,.T.);
#11293=EDGE_CURVE('',#8964,#8962,#1803,.T.);
#11294=EDGE_CURVE('',#8965,#8964,#1804,.T.);
#11295=EDGE_CURVE('',#8963,#8966,#1805,.T.);
#11296=EDGE_CURVE('',#8966,#8965,#1806,.T.);
#11297=EDGE_CURVE('',#8967,#8965,#1807,.T.);
#11298=EDGE_CURVE('',#8966,#8968,#1808,.T.);
#11299=EDGE_CURVE('',#8968,#8967,#1809,.T.);
#11300=EDGE_CURVE('',#8969,#8967,#1810,.T.);
#11301=EDGE_CURVE('',#8968,#8970,#1811,.T.);
#11302=EDGE_CURVE('',#8970,#8969,#1812,.T.);
#11303=EDGE_CURVE('',#8971,#8969,#1813,.T.);
#11304=EDGE_CURVE('',#8970,#8972,#1814,.T.);
#11305=EDGE_CURVE('',#8972,#8971,#1815,.T.);
#11306=EDGE_CURVE('',#8960,#8971,#1816,.T.);
#11307=EDGE_CURVE('',#8972,#8957,#1817,.T.);
#11308=EDGE_CURVE('',#8947,#8969,#1818,.T.);
#11309=EDGE_CURVE('',#8946,#8967,#1819,.T.);
#11310=EDGE_CURVE('',#8940,#8971,#1820,.T.);
#11311=EDGE_CURVE('',#8941,#8960,#1821,.T.);
#11312=EDGE_CURVE('',#8942,#8959,#1822,.T.);
#11313=EDGE_CURVE('',#8973,#8973,#7473,.T.);
#11314=EDGE_CURVE('',#8933,#8927,#1823,.T.);
#11315=EDGE_CURVE('',#8974,#8975,#7474,.T.);
#11316=EDGE_CURVE('',#8975,#8976,#1824,.T.);
#11317=EDGE_CURVE('',#8976,#8976,#7475,.T.);
#11318=EDGE_CURVE('',#8975,#8974,#7476,.T.);
#11319=EDGE_CURVE('',#8977,#8977,#7477,.T.);
#11320=EDGE_CURVE('',#8974,#8956,#1825,.T.);
#11321=EDGE_CURVE('',#8978,#8979,#7478,.T.);
#11322=EDGE_CURVE('',#8979,#8977,#1826,.T.);
#11323=EDGE_CURVE('',#8979,#8978,#7479,.T.);
#11324=EDGE_CURVE('',#8980,#8980,#7480,.T.);
#11325=EDGE_CURVE('',#8980,#8978,#1827,.T.);
#11326=EDGE_CURVE('',#8980,#8981,#1828,.T.);
#11327=EDGE_CURVE('',#8981,#8981,#7481,.T.);
#11328=EDGE_CURVE('',#8982,#8982,#7482,.T.);
#11329=EDGE_CURVE('',#8983,#8983,#7483,.T.);
#11330=EDGE_CURVE('',#8983,#8984,#1829,.T.);
#11331=EDGE_CURVE('',#8984,#8984,#7484,.T.);
#11332=EDGE_CURVE('',#8985,#8985,#7485,.T.);
#11333=EDGE_CURVE('',#8973,#8983,#1830,.T.);
#11334=EDGE_CURVE('',#8986,#8987,#7486,.T.);
#11335=EDGE_CURVE('',#8987,#8985,#1831,.T.);
#11336=EDGE_CURVE('',#8987,#8986,#7487,.T.);
#11337=EDGE_CURVE('',#8986,#8988,#1832,.T.);
#11338=EDGE_CURVE('',#8988,#8988,#7488,.T.);
#11339=EDGE_CURVE('',#8951,#8952,#1833,.T.);
#11340=EDGE_CURVE('',#8950,#8953,#1834,.T.);
#11341=EDGE_CURVE('',#8949,#8954,#1835,.T.);
#11342=EDGE_CURVE('',#8948,#8955,#1836,.T.);
#11343=EDGE_CURVE('',#8989,#8989,#7489,.T.);
#11344=EDGE_CURVE('',#8989,#8982,#1837,.T.);
#11345=EDGE_CURVE('',#8945,#8965,#1838,.T.);
#11346=EDGE_CURVE('',#8944,#8964,#1839,.T.);
#11347=EDGE_CURVE('',#8943,#8962,#1840,.T.);
#15300=ORIENTED_EDGE('',*,*,#11208,.F.);
#15301=ORIENTED_EDGE('',*,*,#11209,.F.);
#15302=ORIENTED_EDGE('',*,*,#11210,.F.);
#15303=ORIENTED_EDGE('',*,*,#11211,.F.);
#15304=ORIENTED_EDGE('',*,*,#11212,.F.);
#15305=ORIENTED_EDGE('',*,*,#11213,.F.);
#15306=ORIENTED_EDGE('',*,*,#11214,.F.);
#15307=ORIENTED_EDGE('',*,*,#11215,.F.);
#15308=ORIENTED_EDGE('',*,*,#11216,.F.);
#15309=ORIENTED_EDGE('',*,*,#11209,.T.);
#15310=ORIENTED_EDGE('',*,*,#11217,.F.);
#15311=ORIENTED_EDGE('',*,*,#11218,.F.);
#15312=ORIENTED_EDGE('',*,*,#11219,.F.);
#15313=ORIENTED_EDGE('',*,*,#11220,.F.);
#15314=ORIENTED_EDGE('',*,*,#11221,.F.);
#15315=ORIENTED_EDGE('',*,*,#11222,.F.);
#15316=ORIENTED_EDGE('',*,*,#11223,.F.);
#15317=ORIENTED_EDGE('',*,*,#11224,.F.);
#15318=ORIENTED_EDGE('',*,*,#11225,.F.);
#15319=ORIENTED_EDGE('',*,*,#11218,.T.);
#15320=ORIENTED_EDGE('',*,*,#11226,.F.);
#15321=ORIENTED_EDGE('',*,*,#11227,.F.);
#15322=ORIENTED_EDGE('',*,*,#11228,.F.);
#15323=ORIENTED_EDGE('',*,*,#11229,.F.);
#15324=ORIENTED_EDGE('',*,*,#11230,.F.);
#15325=ORIENTED_EDGE('',*,*,#11231,.F.);
#15326=ORIENTED_EDGE('',*,*,#11232,.F.);
#15327=ORIENTED_EDGE('',*,*,#11233,.F.);
#15328=ORIENTED_EDGE('',*,*,#11234,.F.);
#15329=ORIENTED_EDGE('',*,*,#11227,.T.);
#15330=ORIENTED_EDGE('',*,*,#11235,.F.);
#15331=ORIENTED_EDGE('',*,*,#11236,.F.);
#15332=ORIENTED_EDGE('',*,*,#11237,.F.);
#15333=ORIENTED_EDGE('',*,*,#11238,.F.);
#15334=ORIENTED_EDGE('',*,*,#11239,.F.);
#15335=ORIENTED_EDGE('',*,*,#11240,.F.);
#15336=ORIENTED_EDGE('',*,*,#11241,.F.);
#15337=ORIENTED_EDGE('',*,*,#11242,.F.);
#15338=ORIENTED_EDGE('',*,*,#11243,.F.);
#15339=ORIENTED_EDGE('',*,*,#11236,.T.);
#15340=ORIENTED_EDGE('',*,*,#11244,.F.);
#15341=ORIENTED_EDGE('',*,*,#11245,.F.);
#15342=ORIENTED_EDGE('',*,*,#11246,.F.);
#15343=ORIENTED_EDGE('',*,*,#11213,.T.);
#15344=ORIENTED_EDGE('',*,*,#11247,.F.);
#15345=ORIENTED_EDGE('',*,*,#11248,.F.);
#15346=ORIENTED_EDGE('',*,*,#11249,.F.);
#15347=ORIENTED_EDGE('',*,*,#11222,.T.);
#15348=ORIENTED_EDGE('',*,*,#11250,.F.);
#15349=ORIENTED_EDGE('',*,*,#11251,.F.);
#15350=ORIENTED_EDGE('',*,*,#11252,.F.);
#15351=ORIENTED_EDGE('',*,*,#11231,.T.);
#15352=ORIENTED_EDGE('',*,*,#11253,.F.);
#15353=ORIENTED_EDGE('',*,*,#11254,.F.);
#15354=ORIENTED_EDGE('',*,*,#11255,.F.);
#15355=ORIENTED_EDGE('',*,*,#11240,.T.);
#15356=ORIENTED_EDGE('',*,*,#11211,.T.);
#15357=ORIENTED_EDGE('',*,*,#11256,.F.);
#15358=ORIENTED_EDGE('',*,*,#11248,.T.);
#15359=ORIENTED_EDGE('',*,*,#11257,.T.);
#15360=ORIENTED_EDGE('',*,*,#11210,.T.);
#15361=ORIENTED_EDGE('',*,*,#11216,.T.);
#15362=ORIENTED_EDGE('',*,*,#11258,.T.);
#15363=ORIENTED_EDGE('',*,*,#11223,.T.);
#15364=ORIENTED_EDGE('',*,*,#11249,.T.);
#15365=ORIENTED_EDGE('',*,*,#11256,.T.);
#15366=ORIENTED_EDGE('',*,*,#11220,.T.);
#15367=ORIENTED_EDGE('',*,*,#11259,.F.);
#15368=ORIENTED_EDGE('',*,*,#11251,.T.);
#15369=ORIENTED_EDGE('',*,*,#11260,.T.);
#15370=ORIENTED_EDGE('',*,*,#11219,.T.);
#15371=ORIENTED_EDGE('',*,*,#11225,.T.);
#15372=ORIENTED_EDGE('',*,*,#11261,.T.);
#15373=ORIENTED_EDGE('',*,*,#11232,.T.);
#15374=ORIENTED_EDGE('',*,*,#11252,.T.);
#15375=ORIENTED_EDGE('',*,*,#11259,.T.);
#15376=ORIENTED_EDGE('',*,*,#11229,.T.);
#15377=ORIENTED_EDGE('',*,*,#11262,.F.);
#15378=ORIENTED_EDGE('',*,*,#11254,.T.);
#15379=ORIENTED_EDGE('',*,*,#11263,.T.);
#15380=ORIENTED_EDGE('',*,*,#11244,.T.);
#15381=ORIENTED_EDGE('',*,*,#11212,.T.);
#15382=ORIENTED_EDGE('',*,*,#11208,.T.);
#15383=ORIENTED_EDGE('',*,*,#11257,.F.);
#15384=ORIENTED_EDGE('',*,*,#11247,.T.);
#15385=ORIENTED_EDGE('',*,*,#11221,.T.);
#15386=ORIENTED_EDGE('',*,*,#11217,.T.);
#15387=ORIENTED_EDGE('',*,*,#11260,.F.);
#15388=ORIENTED_EDGE('',*,*,#11250,.T.);
#15389=ORIENTED_EDGE('',*,*,#11230,.T.);
#15390=ORIENTED_EDGE('',*,*,#11226,.T.);
#15391=ORIENTED_EDGE('',*,*,#11263,.F.);
#15392=ORIENTED_EDGE('',*,*,#11253,.T.);
#15393=ORIENTED_EDGE('',*,*,#11239,.T.);
#15394=ORIENTED_EDGE('',*,*,#11235,.T.);
#15395=ORIENTED_EDGE('',*,*,#11264,.F.);
#15396=ORIENTED_EDGE('',*,*,#11265,.T.);
#15397=ORIENTED_EDGE('',*,*,#11266,.T.);
#15398=ORIENTED_EDGE('',*,*,#11267,.T.);
#15399=ORIENTED_EDGE('',*,*,#11268,.T.);
#15400=ORIENTED_EDGE('',*,*,#11269,.T.);
#15401=ORIENTED_EDGE('',*,*,#11270,.T.);
#15402=ORIENTED_EDGE('',*,*,#11271,.T.);
#15403=ORIENTED_EDGE('',*,*,#11272,.T.);
#15404=ORIENTED_EDGE('',*,*,#11273,.T.);
#15405=ORIENTED_EDGE('',*,*,#11274,.T.);
#15406=ORIENTED_EDGE('',*,*,#11275,.T.);
#15407=ORIENTED_EDGE('',*,*,#11276,.T.);
#15408=ORIENTED_EDGE('',*,*,#11228,.T.);
#15409=ORIENTED_EDGE('',*,*,#11234,.T.);
#15410=ORIENTED_EDGE('',*,*,#11277,.T.);
#15411=ORIENTED_EDGE('',*,*,#11241,.T.);
#15412=ORIENTED_EDGE('',*,*,#11255,.T.);
#15413=ORIENTED_EDGE('',*,*,#11262,.T.);
#15414=ORIENTED_EDGE('',*,*,#11215,.T.);
#15415=ORIENTED_EDGE('',*,*,#11278,.F.);
#15416=ORIENTED_EDGE('',*,*,#11242,.T.);
#15417=ORIENTED_EDGE('',*,*,#11277,.F.);
#15418=ORIENTED_EDGE('',*,*,#11233,.T.);
#15419=ORIENTED_EDGE('',*,*,#11261,.F.);
#15420=ORIENTED_EDGE('',*,*,#11224,.T.);
#15421=ORIENTED_EDGE('',*,*,#11258,.F.);
#15422=ORIENTED_EDGE('',*,*,#11279,.T.);
#15423=ORIENTED_EDGE('',*,*,#11280,.T.);
#15424=ORIENTED_EDGE('',*,*,#11281,.T.);
#15425=ORIENTED_EDGE('',*,*,#11282,.T.);
#15426=ORIENTED_EDGE('',*,*,#11283,.T.);
#15427=ORIENTED_EDGE('',*,*,#11284,.T.);
#15428=ORIENTED_EDGE('',*,*,#11285,.T.);
#15429=ORIENTED_EDGE('',*,*,#11286,.T.);
#15430=ORIENTED_EDGE('',*,*,#11287,.F.);
#15431=ORIENTED_EDGE('',*,*,#11288,.T.);
#15432=ORIENTED_EDGE('',*,*,#11289,.T.);
#15433=ORIENTED_EDGE('',*,*,#11290,.T.);
#15434=ORIENTED_EDGE('',*,*,#11285,.F.);
#15435=ORIENTED_EDGE('',*,*,#11291,.T.);
#15436=ORIENTED_EDGE('',*,*,#11292,.T.);
#15437=ORIENTED_EDGE('',*,*,#11293,.T.);
#15438=ORIENTED_EDGE('',*,*,#11289,.F.);
#15439=ORIENTED_EDGE('',*,*,#11294,.T.);
#15440=ORIENTED_EDGE('',*,*,#11292,.F.);
#15441=ORIENTED_EDGE('',*,*,#11295,.T.);
#15442=ORIENTED_EDGE('',*,*,#11296,.T.);
#15443=ORIENTED_EDGE('',*,*,#11297,.T.);
#15444=ORIENTED_EDGE('',*,*,#11296,.F.);
#15445=ORIENTED_EDGE('',*,*,#11298,.T.);
#15446=ORIENTED_EDGE('',*,*,#11299,.T.);
#15447=ORIENTED_EDGE('',*,*,#11300,.T.);
#15448=ORIENTED_EDGE('',*,*,#11299,.F.);
#15449=ORIENTED_EDGE('',*,*,#11301,.T.);
#15450=ORIENTED_EDGE('',*,*,#11302,.T.);
#15451=ORIENTED_EDGE('',*,*,#11303,.T.);
#15452=ORIENTED_EDGE('',*,*,#11302,.F.);
#15453=ORIENTED_EDGE('',*,*,#11304,.T.);
#15454=ORIENTED_EDGE('',*,*,#11305,.T.);
#15455=ORIENTED_EDGE('',*,*,#11306,.T.);
#15456=ORIENTED_EDGE('',*,*,#11305,.F.);
#15457=ORIENTED_EDGE('',*,*,#11307,.T.);
#15458=ORIENTED_EDGE('',*,*,#11287,.T.);
#15459=ORIENTED_EDGE('',*,*,#11300,.F.);
#15460=ORIENTED_EDGE('',*,*,#11308,.F.);
#15461=ORIENTED_EDGE('',*,*,#11271,.F.);
#15462=ORIENTED_EDGE('',*,*,#11309,.T.);
#15463=ORIENTED_EDGE('',*,*,#11303,.F.);
#15464=ORIENTED_EDGE('',*,*,#11310,.F.);
#15465=ORIENTED_EDGE('',*,*,#11272,.F.);
#15466=ORIENTED_EDGE('',*,*,#11308,.T.);
#15467=ORIENTED_EDGE('',*,*,#11306,.F.);
#15468=ORIENTED_EDGE('',*,*,#11311,.F.);
#15469=ORIENTED_EDGE('',*,*,#11265,.F.);
#15470=ORIENTED_EDGE('',*,*,#11310,.T.);
#15471=ORIENTED_EDGE('',*,*,#11286,.F.);
#15472=ORIENTED_EDGE('',*,*,#11312,.F.);
#15473=ORIENTED_EDGE('',*,*,#11266,.F.);
#15474=ORIENTED_EDGE('',*,*,#11311,.T.);
#15475=ORIENTED_EDGE('',*,*,#11284,.F.);
#15476=ORIENTED_EDGE('',*,*,#11307,.F.);
#15477=ORIENTED_EDGE('',*,*,#11304,.F.);
#15478=ORIENTED_EDGE('',*,*,#11301,.F.);
#15479=ORIENTED_EDGE('',*,*,#11298,.F.);
#15480=ORIENTED_EDGE('',*,*,#11295,.F.);
#15481=ORIENTED_EDGE('',*,*,#11291,.F.);
#15482=ORIENTED_EDGE('',*,*,#11288,.F.);
#15483=ORIENTED_EDGE('',*,*,#11313,.F.);
#15484=ORIENTED_EDGE('',*,*,#11246,.T.);
#15485=ORIENTED_EDGE('',*,*,#11314,.T.);
#15486=ORIENTED_EDGE('',*,*,#11237,.T.);
#15487=ORIENTED_EDGE('',*,*,#11243,.T.);
#15488=ORIENTED_EDGE('',*,*,#11278,.T.);
#15489=ORIENTED_EDGE('',*,*,#11214,.T.);
#15490=ORIENTED_EDGE('',*,*,#11315,.T.);
#15491=ORIENTED_EDGE('',*,*,#11316,.T.);
#15492=ORIENTED_EDGE('',*,*,#11317,.T.);
#15493=ORIENTED_EDGE('',*,*,#11316,.F.);
#15494=ORIENTED_EDGE('',*,*,#11318,.T.);
#15495=ORIENTED_EDGE('',*,*,#11317,.F.);
#15496=ORIENTED_EDGE('',*,*,#11319,.F.);
#15497=ORIENTED_EDGE('',*,*,#11315,.F.);
#15498=ORIENTED_EDGE('',*,*,#11320,.T.);
#15499=ORIENTED_EDGE('',*,*,#11283,.F.);
#15500=ORIENTED_EDGE('',*,*,#11320,.F.);
#15501=ORIENTED_EDGE('',*,*,#11318,.F.);
#15502=ORIENTED_EDGE('',*,*,#11321,.T.);
#15503=ORIENTED_EDGE('',*,*,#11322,.T.);
#15504=ORIENTED_EDGE('',*,*,#11319,.T.);
#15505=ORIENTED_EDGE('',*,*,#11322,.F.);
#15506=ORIENTED_EDGE('',*,*,#11323,.T.);
#15507=ORIENTED_EDGE('',*,*,#11324,.F.);
#15508=ORIENTED_EDGE('',*,*,#11325,.T.);
#15509=ORIENTED_EDGE('',*,*,#11323,.F.);
#15510=ORIENTED_EDGE('',*,*,#11321,.F.);
#15511=ORIENTED_EDGE('',*,*,#11325,.F.);
#15512=ORIENTED_EDGE('',*,*,#11324,.T.);
#15513=ORIENTED_EDGE('',*,*,#11326,.T.);
#15514=ORIENTED_EDGE('',*,*,#11327,.T.);
#15515=ORIENTED_EDGE('',*,*,#11326,.F.);
#15516=ORIENTED_EDGE('',*,*,#11328,.F.);
#15517=ORIENTED_EDGE('',*,*,#11327,.F.);
#15518=ORIENTED_EDGE('',*,*,#11329,.T.);
#15519=ORIENTED_EDGE('',*,*,#11330,.T.);
#15520=ORIENTED_EDGE('',*,*,#11331,.T.);
#15521=ORIENTED_EDGE('',*,*,#11330,.F.);
#15522=ORIENTED_EDGE('',*,*,#11331,.F.);
#15523=ORIENTED_EDGE('',*,*,#11332,.F.);
#15524=ORIENTED_EDGE('',*,*,#11313,.T.);
#15525=ORIENTED_EDGE('',*,*,#11333,.T.);
#15526=ORIENTED_EDGE('',*,*,#11329,.F.);
#15527=ORIENTED_EDGE('',*,*,#11333,.F.);
#15528=ORIENTED_EDGE('',*,*,#11334,.T.);
#15529=ORIENTED_EDGE('',*,*,#11335,.T.);
#15530=ORIENTED_EDGE('',*,*,#11332,.T.);
#15531=ORIENTED_EDGE('',*,*,#11335,.F.);
#15532=ORIENTED_EDGE('',*,*,#11336,.T.);
#15533=ORIENTED_EDGE('',*,*,#11334,.F.);
#15534=ORIENTED_EDGE('',*,*,#11337,.T.);
#15535=ORIENTED_EDGE('',*,*,#11338,.T.);
#15536=ORIENTED_EDGE('',*,*,#11337,.F.);
#15537=ORIENTED_EDGE('',*,*,#11336,.F.);
#15538=ORIENTED_EDGE('',*,*,#11276,.F.);
#15539=ORIENTED_EDGE('',*,*,#11339,.T.);
#15540=ORIENTED_EDGE('',*,*,#11279,.F.);
#15541=ORIENTED_EDGE('',*,*,#11339,.F.);
#15542=ORIENTED_EDGE('',*,*,#11275,.F.);
#15543=ORIENTED_EDGE('',*,*,#11340,.T.);
#15544=ORIENTED_EDGE('',*,*,#11280,.F.);
#15545=ORIENTED_EDGE('',*,*,#11340,.F.);
#15546=ORIENTED_EDGE('',*,*,#11274,.F.);
#15547=ORIENTED_EDGE('',*,*,#11341,.T.);
#15548=ORIENTED_EDGE('',*,*,#11281,.F.);
#15549=ORIENTED_EDGE('',*,*,#11341,.F.);
#15550=ORIENTED_EDGE('',*,*,#11273,.F.);
#15551=ORIENTED_EDGE('',*,*,#11342,.T.);
#15552=ORIENTED_EDGE('',*,*,#11282,.F.);
#15553=ORIENTED_EDGE('',*,*,#11342,.F.);
#15554=ORIENTED_EDGE('',*,*,#11343,.F.);
#15555=ORIENTED_EDGE('',*,*,#11344,.T.);
#15556=ORIENTED_EDGE('',*,*,#11328,.T.);
#15557=ORIENTED_EDGE('',*,*,#11344,.F.);
#15558=ORIENTED_EDGE('',*,*,#11338,.F.);
#15559=ORIENTED_EDGE('',*,*,#11343,.T.);
#15560=ORIENTED_EDGE('',*,*,#11297,.F.);
#15561=ORIENTED_EDGE('',*,*,#11309,.F.);
#15562=ORIENTED_EDGE('',*,*,#11270,.F.);
#15563=ORIENTED_EDGE('',*,*,#11345,.T.);
#15564=ORIENTED_EDGE('',*,*,#11294,.F.);
#15565=ORIENTED_EDGE('',*,*,#11345,.F.);
#15566=ORIENTED_EDGE('',*,*,#11269,.F.);
#15567=ORIENTED_EDGE('',*,*,#11346,.T.);
#15568=ORIENTED_EDGE('',*,*,#11293,.F.);
#15569=ORIENTED_EDGE('',*,*,#11346,.F.);
#15570=ORIENTED_EDGE('',*,*,#11268,.F.);
#15571=ORIENTED_EDGE('',*,*,#11347,.T.);
#15572=ORIENTED_EDGE('',*,*,#11290,.F.);
#15573=ORIENTED_EDGE('',*,*,#11347,.F.);
#15574=ORIENTED_EDGE('',*,*,#11267,.F.);
#15575=ORIENTED_EDGE('',*,*,#11312,.T.);
#15576=ORIENTED_EDGE('',*,*,#11245,.T.);
#15577=ORIENTED_EDGE('',*,*,#11264,.T.);
#15578=ORIENTED_EDGE('',*,*,#11238,.T.);
#15579=ORIENTED_EDGE('',*,*,#11314,.F.);
#18968=ADVANCED_FACE('',(#5252),#4504,.T.);
#18969=ADVANCED_FACE('',(#5253),#4505,.T.);
#18970=ADVANCED_FACE('',(#5254),#4506,.T.);
#18971=ADVANCED_FACE('',(#5255),#4507,.T.);
#18972=ADVANCED_FACE('',(#5256),#4508,.T.);
#18973=ADVANCED_FACE('',(#5257),#4509,.T.);
#18974=ADVANCED_FACE('',(#5258),#4510,.T.);
#18975=ADVANCED_FACE('',(#5259),#4511,.T.);
#18976=ADVANCED_FACE('',(#5260),#4512,.T.);
#18977=ADVANCED_FACE('',(#5261),#4513,.T.);
#18978=ADVANCED_FACE('',(#5262),#4514,.T.);
#18979=ADVANCED_FACE('',(#5263),#4515,.T.);
#18980=ADVANCED_FACE('',(#5264),#816,.T.);
#18981=ADVANCED_FACE('',(#5265),#817,.T.);
#18982=ADVANCED_FACE('',(#5266),#818,.T.);
#18983=ADVANCED_FACE('',(#5267),#819,.T.);
#18984=ADVANCED_FACE('',(#5268),#820,.T.);
#18985=ADVANCED_FACE('',(#5269,#519,#520,#521,#522,#523),#821,.F.);
#18986=ADVANCED_FACE('',(#5270),#822,.T.);
#18987=ADVANCED_FACE('',(#5271,#524,#525,#526,#527,#528),#823,.T.);
#18988=ADVANCED_FACE('',(#5272),#824,.T.);
#18989=ADVANCED_FACE('',(#5273),#825,.T.);
#18990=ADVANCED_FACE('',(#5274),#826,.T.);
#18991=ADVANCED_FACE('',(#5275),#827,.T.);
#18992=ADVANCED_FACE('',(#5276),#828,.T.);
#18993=ADVANCED_FACE('',(#5277),#829,.T.);
#18994=ADVANCED_FACE('',(#5278),#830,.T.);
#18995=ADVANCED_FACE('',(#5279),#831,.T.);
#18996=ADVANCED_FACE('',(#5280),#832,.F.);
#18997=ADVANCED_FACE('',(#5281),#833,.F.);
#18998=ADVANCED_FACE('',(#5282),#834,.F.);
#18999=ADVANCED_FACE('',(#5283),#835,.F.);
#19000=ADVANCED_FACE('',(#5284,#529),#836,.T.);
#19001=ADVANCED_FACE('',(#5285),#837,.T.);
#19002=ADVANCED_FACE('',(#5286),#180,.T.);
#19003=ADVANCED_FACE('',(#5287,#530),#838,.T.);
#19004=ADVANCED_FACE('',(#5288),#4516,.T.);
#19005=ADVANCED_FACE('',(#5289),#181,.F.);
#19006=ADVANCED_FACE('',(#5290),#4517,.F.);
#19007=ADVANCED_FACE('',(#5291),#182,.F.);
#19008=ADVANCED_FACE('',(#5292,#531),#839,.T.);
#19009=ADVANCED_FACE('',(#5293),#183,.T.);
#19010=ADVANCED_FACE('',(#5294,#532),#840,.T.);
#19011=ADVANCED_FACE('',(#5295),#4518,.T.);
#19012=ADVANCED_FACE('',(#5296),#184,.F.);
#19013=ADVANCED_FACE('',(#5297),#4519,.F.);
#19014=ADVANCED_FACE('',(#5298),#4520,.F.);
#19015=ADVANCED_FACE('',(#5299),#4521,.F.);
#19016=ADVANCED_FACE('',(#5300),#4522,.F.);
#19017=ADVANCED_FACE('',(#5301),#4523,.F.);
#19018=ADVANCED_FACE('',(#5302),#4524,.F.);
#19019=ADVANCED_FACE('',(#5303,#533),#841,.T.);
#19020=ADVANCED_FACE('',(#5304),#842,.F.);
#19021=ADVANCED_FACE('',(#5305),#843,.F.);
#19022=ADVANCED_FACE('',(#5306),#844,.F.);
#19023=ADVANCED_FACE('',(#5307),#845,.F.);
#19024=ADVANCED_FACE('',(#5308),#846,.T.);
#19565=CLOSED_SHELL('',(#18968,#18969,#18970,#18971,#18972,#18973,#18974,
#18975,#18976,#18977,#18978,#18979,#18980,#18981,#18982,#18983,#18984,#18985,
#18986,#18987,#18988,#18989,#18990,#18991,#18992,#18993,#18994,#18995,#18996,
#18997,#18998,#18999,#19000,#19001,#19002,#19003,#19004,#19005,#19006,#19007,
#19008,#19009,#19010,#19011,#19012,#19013,#19014,#19015,#19016,#19017,#19018,
#19019,#19020,#19021,#19022,#19023,#19024));
#20965=AXIS2_PLACEMENT_3D('',#31308,#24970,#24971);
#20966=AXIS2_PLACEMENT_3D('',#31309,#24972,#24973);
#20967=AXIS2_PLACEMENT_3D('',#31312,#24974,#24975);
#20968=AXIS2_PLACEMENT_3D('',#31316,#24977,#24978);
#20969=AXIS2_PLACEMENT_3D('',#31317,#24979,#24980);
#20970=AXIS2_PLACEMENT_3D('',#31318,#24981,#24982);
#20971=AXIS2_PLACEMENT_3D('',#31320,#24983,#24984);
#20972=AXIS2_PLACEMENT_3D('',#31324,#24986,#24987);
#20973=AXIS2_PLACEMENT_3D('',#31326,#24988,#24989);
#20974=AXIS2_PLACEMENT_3D('',#31327,#24990,#24991);
#20975=AXIS2_PLACEMENT_3D('',#31328,#24992,#24993);
#20976=AXIS2_PLACEMENT_3D('',#31331,#24994,#24995);
#20977=AXIS2_PLACEMENT_3D('',#31335,#24997,#24998);
#20978=AXIS2_PLACEMENT_3D('',#31336,#24999,#25000);
#20979=AXIS2_PLACEMENT_3D('',#31337,#25001,#25002);
#20980=AXIS2_PLACEMENT_3D('',#31339,#25003,#25004);
#20981=AXIS2_PLACEMENT_3D('',#31343,#25006,#25007);
#20982=AXIS2_PLACEMENT_3D('',#31345,#25008,#25009);
#20983=AXIS2_PLACEMENT_3D('',#31346,#25010,#25011);
#20984=AXIS2_PLACEMENT_3D('',#31347,#25012,#25013);
#20985=AXIS2_PLACEMENT_3D('',#31350,#25014,#25015);
#20986=AXIS2_PLACEMENT_3D('',#31354,#25017,#25018);
#20987=AXIS2_PLACEMENT_3D('',#31355,#25019,#25020);
#20988=AXIS2_PLACEMENT_3D('',#31356,#25021,#25022);
#20989=AXIS2_PLACEMENT_3D('',#31358,#25023,#25024);
#20990=AXIS2_PLACEMENT_3D('',#31362,#25026,#25027);
#20991=AXIS2_PLACEMENT_3D('',#31364,#25028,#25029);
#20992=AXIS2_PLACEMENT_3D('',#31365,#25030,#25031);
#20993=AXIS2_PLACEMENT_3D('',#31366,#25032,#25033);
#20994=AXIS2_PLACEMENT_3D('',#31369,#25034,#25035);
#20995=AXIS2_PLACEMENT_3D('',#31373,#25037,#25038);
#20996=AXIS2_PLACEMENT_3D('',#31374,#25039,#25040);
#20997=AXIS2_PLACEMENT_3D('',#31375,#25041,#25042);
#20998=AXIS2_PLACEMENT_3D('',#31377,#25043,#25044);
#20999=AXIS2_PLACEMENT_3D('',#31381,#25046,#25047);
#21000=AXIS2_PLACEMENT_3D('',#31383,#25048,#25049);
#21001=AXIS2_PLACEMENT_3D('',#31384,#25050,#25051);
#21002=AXIS2_PLACEMENT_3D('',#31385,#25052,#25053);
#21003=AXIS2_PLACEMENT_3D('',#31387,#25054,#25055);
#21004=AXIS2_PLACEMENT_3D('',#31389,#25056,#25057);
#21005=AXIS2_PLACEMENT_3D('',#31390,#25058,#25059);
#21006=AXIS2_PLACEMENT_3D('',#31391,#25060,#25061);
#21007=AXIS2_PLACEMENT_3D('',#31393,#25062,#25063);
#21008=AXIS2_PLACEMENT_3D('',#31395,#25064,#25065);
#21009=AXIS2_PLACEMENT_3D('',#31396,#25066,#25067);
#21010=AXIS2_PLACEMENT_3D('',#31397,#25068,#25069);
#21011=AXIS2_PLACEMENT_3D('',#31399,#25070,#25071);
#21012=AXIS2_PLACEMENT_3D('',#31401,#25072,#25073);
#21013=AXIS2_PLACEMENT_3D('',#31402,#25074,#25075);
#21014=AXIS2_PLACEMENT_3D('',#31403,#25076,#25077);
#21015=AXIS2_PLACEMENT_3D('',#31405,#25078,#25079);
#21016=AXIS2_PLACEMENT_3D('',#31407,#25080,#25081);
#21017=AXIS2_PLACEMENT_3D('',#31408,#25082,#25083);
#21018=AXIS2_PLACEMENT_3D('',#31409,#25084,#25085);
#21019=AXIS2_PLACEMENT_3D('',#31412,#25088,#25089);
#21020=AXIS2_PLACEMENT_3D('',#31414,#25091,#25092);
#21021=AXIS2_PLACEMENT_3D('',#31417,#25095,#25096);
#21022=AXIS2_PLACEMENT_3D('',#31419,#25098,#25099);
#21023=AXIS2_PLACEMENT_3D('',#31422,#25102,#25103);
#21024=AXIS2_PLACEMENT_3D('',#31441,#25113,#25114);
#21025=AXIS2_PLACEMENT_3D('',#31443,#25115,#25116);
#21026=AXIS2_PLACEMENT_3D('',#31445,#25117,#25118);
#21027=AXIS2_PLACEMENT_3D('',#31447,#25119,#25120);
#21028=AXIS2_PLACEMENT_3D('',#31448,#25121,#25122);
#21029=AXIS2_PLACEMENT_3D('',#31450,#25124,#25125);
#21030=AXIS2_PLACEMENT_3D('',#31453,#25127,#25128);
#21031=AXIS2_PLACEMENT_3D('',#31455,#25129,#25130);
#21032=AXIS2_PLACEMENT_3D('',#31457,#25131,#25132);
#21033=AXIS2_PLACEMENT_3D('',#31459,#25133,#25134);
#21034=AXIS2_PLACEMENT_3D('',#31461,#25135,#25136);
#21035=AXIS2_PLACEMENT_3D('',#31462,#25137,#25138);
#21036=AXIS2_PLACEMENT_3D('',#31471,#25143,#25144);
#21037=AXIS2_PLACEMENT_3D('',#31477,#25148,#25149);
#21038=AXIS2_PLACEMENT_3D('',#31483,#25153,#25154);
#21039=AXIS2_PLACEMENT_3D('',#31489,#25158,#25159);
#21040=AXIS2_PLACEMENT_3D('',#31495,#25163,#25164);
#21041=AXIS2_PLACEMENT_3D('',#31501,#25168,#25169);
#21042=AXIS2_PLACEMENT_3D('',#31507,#25173,#25174);
#21043=AXIS2_PLACEMENT_3D('',#31510,#25177,#25178);
#21044=AXIS2_PLACEMENT_3D('',#31513,#25181,#25182);
#21045=AXIS2_PLACEMENT_3D('',#31515,#25184,#25185);
#21046=AXIS2_PLACEMENT_3D('',#31517,#25187,#25188);
#21047=AXIS2_PLACEMENT_3D('',#31519,#25190,#25191);
#21048=AXIS2_PLACEMENT_3D('',#31521,#25192,#25193);
#21049=AXIS2_PLACEMENT_3D('',#31522,#25194,#25195);
#21050=AXIS2_PLACEMENT_3D('',#31524,#25197,#25198);
#21051=AXIS2_PLACEMENT_3D('',#31527,#25199,#25200);
#21052=AXIS2_PLACEMENT_3D('',#31530,#25202,#25203);
#21053=AXIS2_PLACEMENT_3D('',#31531,#25204,#25205);
#21054=AXIS2_PLACEMENT_3D('',#31532,#25206,#25207);
#21055=AXIS2_PLACEMENT_3D('',#31534,#25208,#25209);
#21056=AXIS2_PLACEMENT_3D('',#31535,#25210,#25211);
#21057=AXIS2_PLACEMENT_3D('',#31537,#25213,#25214);
#21058=AXIS2_PLACEMENT_3D('',#31540,#25215,#25216);
#21059=AXIS2_PLACEMENT_3D('',#31542,#25218,#25219);
#21060=AXIS2_PLACEMENT_3D('',#31543,#25220,#25221);
#21061=AXIS2_PLACEMENT_3D('',#31545,#25222,#25223);
#21062=AXIS2_PLACEMENT_3D('',#31547,#25225,#25226);
#21063=AXIS2_PLACEMENT_3D('',#31550,#25228,#25229);
#21064=AXIS2_PLACEMENT_3D('',#31551,#25230,#25231);
#21065=AXIS2_PLACEMENT_3D('',#31553,#25232,#25233);
#21066=AXIS2_PLACEMENT_3D('',#31554,#25234,#25235);
#21067=AXIS2_PLACEMENT_3D('',#31556,#25236,#25237);
#21068=AXIS2_PLACEMENT_3D('',#31559,#25239,#25240);
#21069=AXIS2_PLACEMENT_3D('',#31560,#25241,#25242);
#21070=AXIS2_PLACEMENT_3D('',#31562,#25243,#25244);
#21071=AXIS2_PLACEMENT_3D('',#31563,#25245,#25246);
#21072=AXIS2_PLACEMENT_3D('',#31565,#25248,#25249);
#21073=AXIS2_PLACEMENT_3D('',#31568,#25250,#25251);
#21074=AXIS2_PLACEMENT_3D('',#31570,#25253,#25254);
#21075=AXIS2_PLACEMENT_3D('',#31571,#25255,#25256);
#21076=AXIS2_PLACEMENT_3D('',#31574,#25258,#25259);
#21077=AXIS2_PLACEMENT_3D('',#31575,#25260,#25261);
#21078=AXIS2_PLACEMENT_3D('',#31577,#25263,#25264);
#21079=AXIS2_PLACEMENT_3D('',#31579,#25266,#25267);
#21080=AXIS2_PLACEMENT_3D('',#31581,#25269,#25270);
#21081=AXIS2_PLACEMENT_3D('',#31583,#25272,#25273);
#21082=AXIS2_PLACEMENT_3D('',#31585,#25274,#25275);
#21083=AXIS2_PLACEMENT_3D('',#31587,#25277,#25278);
#21084=AXIS2_PLACEMENT_3D('',#31588,#25279,#25280);
#21085=AXIS2_PLACEMENT_3D('',#31590,#25282,#25283);
#21086=AXIS2_PLACEMENT_3D('',#31592,#25285,#25286);
#21087=AXIS2_PLACEMENT_3D('',#31594,#25288,#25289);
#21088=AXIS2_PLACEMENT_3D('',#31595,#25290,#25291);
#24970=DIRECTION('axis',(0.,0.,1.));
#24971=DIRECTION('refdir',(1.,0.,0.));
#24972=DIRECTION('center_axis',(0.,-1.,0.));
#24973=DIRECTION('ref_axis',(0.560568426942125,0.,0.828108108108858));
#24974=DIRECTION('center_axis',(0.,-1.,0.));
#24975=DIRECTION('ref_axis',(0.560568426942125,0.,0.828108108108858));
#24976=DIRECTION('',(0.,-1.,0.));
#24977=DIRECTION('center_axis',(0.,0.713250449154181,0.700909264299851));
#24978=DIRECTION('ref_axis',(9.89833838717548E-17,-0.700909264299851,0.713250449154181));
#24979=DIRECTION('center_axis',(0.,0.0174524064372833,0.999847695156391));
#24980=DIRECTION('ref_axis',(1.21100396635998E-18,-0.999847695156391,0.0174524064372833));
#24981=DIRECTION('center_axis',(0.,-1.,0.));
#24982=DIRECTION('ref_axis',(0.828108108108418,0.,0.560568426942775));
#24983=DIRECTION('center_axis',(0.,-1.,0.));
#24984=DIRECTION('ref_axis',(0.828108108108418,0.,0.560568426942775));
#24985=DIRECTION('',(0.,-1.,0.));
#24986=DIRECTION('center_axis',(0.700909264299845,0.713250449154187,0.));
#24987=DIRECTION('ref_axis',(0.713250449154187,-0.700909264299845,6.30341947044217E-17));
#24988=DIRECTION('center_axis',(0.,1.,0.));
#24989=DIRECTION('ref_axis',(0.828108108108418,0.,0.560568426942775));
#24990=DIRECTION('center_axis',(0.,0.713250449154181,0.700909264299851));
#24991=DIRECTION('ref_axis',(0.,-0.700909264299851,0.713250449154181));
#24992=DIRECTION('center_axis',(0.,-1.,0.));
#24993=DIRECTION('ref_axis',(-0.828108108108883,0.,0.560568426942087));
#24994=DIRECTION('center_axis',(0.,-1.,0.));
#24995=DIRECTION('ref_axis',(-0.828108108108883,0.,0.560568426942087));
#24996=DIRECTION('',(0.,-1.,0.));
#24997=DIRECTION('center_axis',(-0.700909264299851,0.713250449154181,0.));
#24998=DIRECTION('ref_axis',(-0.713250449154181,-0.700909264299851,0.));
#24999=DIRECTION('center_axis',(-0.999847695156391,0.0174524064372833,0.));
#25000=DIRECTION('ref_axis',(-0.0174524064372833,-0.999847695156391,0.));
#25001=DIRECTION('center_axis',(0.,-1.,0.));
#25002=DIRECTION('ref_axis',(-0.560568426943144,0.,0.828108108108168));
#25003=DIRECTION('center_axis',(0.,-1.,0.));
#25004=DIRECTION('ref_axis',(-0.560568426943144,0.,0.828108108108168));
#25005=DIRECTION('',(0.,-1.,0.));
#25006=DIRECTION('center_axis',(0.,0.713250449154181,0.700909264299851));
#25007=DIRECTION('ref_axis',(6.30341947044626E-17,-0.700909264299851,0.713250449154181));
#25008=DIRECTION('center_axis',(0.,1.,0.));
#25009=DIRECTION('ref_axis',(-0.560568426943144,0.,0.828108108108168));
#25010=DIRECTION('center_axis',(-0.700909264299851,0.713250449154181,0.));
#25011=DIRECTION('ref_axis',(-0.713250449154181,-0.700909264299851,6.30341947044626E-17));
#25012=DIRECTION('center_axis',(0.,-1.,0.));
#25013=DIRECTION('ref_axis',(-0.560568426942121,0.,-0.82810810810886));
#25014=DIRECTION('center_axis',(0.,-1.,0.));
#25015=DIRECTION('ref_axis',(-0.560568426942121,0.,-0.82810810810886));
#25016=DIRECTION('',(0.,-1.,0.));
#25017=DIRECTION('center_axis',(0.,0.713250449154181,-0.700909264299851));
#25018=DIRECTION('ref_axis',(0.,-0.700909264299851,-0.713250449154181));
#25019=DIRECTION('center_axis',(0.,0.0174524064372833,-0.999847695156391));
#25020=DIRECTION('ref_axis',(0.,-0.999847695156391,-0.0174524064372833));
#25021=DIRECTION('center_axis',(0.,-1.,0.));
#25022=DIRECTION('ref_axis',(-0.828108108107798,0.,-0.56056842694369));
#25023=DIRECTION('center_axis',(0.,-1.,0.));
#25024=DIRECTION('ref_axis',(-0.828108108107798,0.,-0.56056842694369));
#25025=DIRECTION('',(0.,-1.,0.));
#25026=DIRECTION('center_axis',(-0.700909264299851,0.713250449154181,0.));
#25027=DIRECTION('ref_axis',(-0.713250449154181,-0.700909264299851,-1.26068389408919E-16));
#25028=DIRECTION('center_axis',(0.,1.,0.));
#25029=DIRECTION('ref_axis',(-0.828108108107798,0.,-0.56056842694369));
#25030=DIRECTION('center_axis',(0.,0.713250449154181,-0.700909264299851));
#25031=DIRECTION('ref_axis',(6.30341947044594E-17,-0.700909264299851,-0.713250449154181));
#25032=DIRECTION('center_axis',(0.,-1.,0.));
#25033=DIRECTION('ref_axis',(0.828108108108829,0.,-0.560568426942167));
#25034=DIRECTION('center_axis',(0.,-1.,0.));
#25035=DIRECTION('ref_axis',(0.828108108108829,0.,-0.560568426942167));
#25036=DIRECTION('',(0.,-1.,0.));
#25037=DIRECTION('center_axis',(0.700909264299845,0.713250449154187,0.));
#25038=DIRECTION('ref_axis',(0.713250449154187,-0.700909264299845,1.48475075808888E-16));
#25039=DIRECTION('center_axis',(0.999847695156391,0.0174524064372833,0.));
#25040=DIRECTION('ref_axis',(0.0174524064372833,-0.999847695156391,0.));
#25041=DIRECTION('center_axis',(0.,-1.,0.));
#25042=DIRECTION('ref_axis',(0.560568426943322,0.,-0.828108108108047));
#25043=DIRECTION('center_axis',(0.,-1.,0.));
#25044=DIRECTION('ref_axis',(0.560568426943322,0.,-0.828108108108047));
#25045=DIRECTION('',(0.,-1.,0.));
#25046=DIRECTION('center_axis',(0.,0.713250449154181,-0.700909264299851));
#25047=DIRECTION('ref_axis',(1.26068389408919E-16,-0.700909264299851,-0.713250449154181));
#25048=DIRECTION('center_axis',(0.,1.,0.));
#25049=DIRECTION('ref_axis',(0.560568426943322,0.,-0.828108108108047));
#25050=DIRECTION('center_axis',(0.700909264299845,0.713250449154187,0.));
#25051=DIRECTION('ref_axis',(0.713250449154187,-0.700909264299845,0.));
#25052=DIRECTION('center_axis',(0.,-1.,0.));
#25053=DIRECTION('ref_axis',(1.,0.,-5.00979119302536E-12));
#25054=DIRECTION('center_axis',(0.,-1.,0.));
#25055=DIRECTION('ref_axis',(1.,0.,-5.00979119302536E-12));
#25056=DIRECTION('center_axis',(0.999847695156391,0.0174524064372833,0.));
#25057=DIRECTION('ref_axis',(0.0174524064372833,-0.999847695156391,-8.74329120666009E-14));
#25058=DIRECTION('center_axis',(0.700909264299845,0.713250449154187,0.));
#25059=DIRECTION('ref_axis',(0.713250449154187,-0.700909264299845,-3.57323581859403E-12));
#25060=DIRECTION('center_axis',(0.,-1.,0.));
#25061=DIRECTION('ref_axis',(5.06308189820828E-12,0.,1.));
#25062=DIRECTION('center_axis',(0.,-1.,0.));
#25063=DIRECTION('ref_axis',(5.06308189820828E-12,0.,1.));
#25064=DIRECTION('center_axis',(0.,0.0174524064372833,0.999847695156391));
#25065=DIRECTION('ref_axis',(8.83629631127828E-14,-0.999847695156391,0.0174524064372833));
#25066=DIRECTION('center_axis',(0.,0.713250449154181,0.700909264299851));
#25067=DIRECTION('ref_axis',(3.61124543800146E-12,-0.700909264299851,0.713250449154181));
#25068=DIRECTION('center_axis',(0.,-1.,0.));
#25069=DIRECTION('ref_axis',(-1.,0.,5.0097911930254E-12));
#25070=DIRECTION('center_axis',(0.,-1.,0.));
#25071=DIRECTION('ref_axis',(-1.,0.,5.0097911930254E-12));
#25072=DIRECTION('center_axis',(-0.999847695156391,0.0174524064372833,0.));
#25073=DIRECTION('ref_axis',(-0.0174524064372833,-0.999847695156391,8.74329120666017E-14));
#25074=DIRECTION('center_axis',(-0.700909264299851,0.713250449154181,0.));
#25075=DIRECTION('ref_axis',(-0.713250449154181,-0.700909264299851,3.57323581859403E-12));
#25076=DIRECTION('center_axis',(0.,-1.,0.));
#25077=DIRECTION('ref_axis',(-4.92541424309684E-12,0.,-1.));
#25078=DIRECTION('center_axis',(0.,-1.,0.));
#25079=DIRECTION('ref_axis',(-4.92541424309684E-12,0.,-1.));
#25080=DIRECTION('center_axis',(0.,0.0174524064372833,-0.999847695156391));
#25081=DIRECTION('ref_axis',(-8.59603312425102E-14,-0.999847695156391,-0.0174524064372833));
#25082=DIRECTION('center_axis',(0.,0.713250449154181,-0.700909264299851));
#25083=DIRECTION('ref_axis',(-3.51305392115922E-12,-0.700909264299851,-0.713250449154181));
#25084=DIRECTION('center_axis',(0.,0.0174524064372833,0.999847695156391));
#25085=DIRECTION('ref_axis',(1.,0.,0.));
#25086=DIRECTION('',(1.,0.,0.));
#25087=DIRECTION('',(1.,0.,0.));
#25088=DIRECTION('center_axis',(0.,0.713250449154181,0.700909264299851));
#25089=DIRECTION('ref_axis',(1.,0.,0.));
#25090=DIRECTION('',(-1.,0.,0.));
#25091=DIRECTION('center_axis',(-0.999847695156391,0.0174524064372833,0.));
#25092=DIRECTION('ref_axis',(0.,0.,1.));
#25093=DIRECTION('',(0.,0.,1.));
#25094=DIRECTION('',(0.,0.,1.));
#25095=DIRECTION('center_axis',(-0.700909264299851,0.713250449154181,0.));
#25096=DIRECTION('ref_axis',(0.,0.,1.));
#25097=DIRECTION('',(0.,0.,-1.));
#25098=DIRECTION('center_axis',(0.,0.0174524064372833,-0.999847695156391));
#25099=DIRECTION('ref_axis',(-1.,0.,0.));
#25100=DIRECTION('',(-1.,0.,0.));
#25101=DIRECTION('',(-1.,0.,0.));
#25102=DIRECTION('center_axis',(0.,1.,0.));
#25103=DIRECTION('ref_axis',(1.,0.,0.));
#25104=DIRECTION('',(0.,0.,-1.));
#25105=DIRECTION('',(0.707106781186548,0.,-0.707106781186548));
#25106=DIRECTION('',(-1.00027490415113E-12,0.,-1.));
#25107=DIRECTION('',(-0.707106781186548,0.,-0.707106781186547));
#25108=DIRECTION('',(-1.,0.,1.00013745207507E-12));
#25109=DIRECTION('',(-0.707106781186547,0.,0.707106781186548));
#25110=DIRECTION('',(1.00013745207507E-12,0.,1.));
#25111=DIRECTION('',(0.707106781186548,0.,0.707106781186548));
#25112=DIRECTION('',(1.,0.,0.));
#25113=DIRECTION('center_axis',(0.,1.,0.));
#25114=DIRECTION('ref_axis',(1.,0.,0.));
#25115=DIRECTION('center_axis',(0.,1.,0.));
#25116=DIRECTION('ref_axis',(1.,0.,0.));
#25117=DIRECTION('center_axis',(0.,1.,0.));
#25118=DIRECTION('ref_axis',(1.,0.,0.));
#25119=DIRECTION('center_axis',(0.,1.,0.));
#25120=DIRECTION('ref_axis',(1.,0.,0.));
#25121=DIRECTION('center_axis',(0.,0.713250449154181,-0.700909264299851));
#25122=DIRECTION('ref_axis',(-1.,0.,0.));
#25123=DIRECTION('',(1.,0.,0.));
#25124=DIRECTION('center_axis',(0.,1.,0.));
#25125=DIRECTION('ref_axis',(1.,0.,0.));
#25126=DIRECTION('',(0.,0.,1.));
#25127=DIRECTION('center_axis',(0.,-1.,0.));
#25128=DIRECTION('ref_axis',(1.,0.,0.));
#25129=DIRECTION('center_axis',(0.,-1.,0.));
#25130=DIRECTION('ref_axis',(1.,0.,0.));
#25131=DIRECTION('center_axis',(0.,-1.,0.));
#25132=DIRECTION('ref_axis',(1.,0.,0.));
#25133=DIRECTION('center_axis',(0.,-1.,0.));
#25134=DIRECTION('ref_axis',(1.,0.,0.));
#25135=DIRECTION('center_axis',(0.,-1.,0.));
#25136=DIRECTION('ref_axis',(1.,0.,0.));
#25137=DIRECTION('center_axis',(-0.707106781186547,-0.707106781186548,1.94386590150466E-16));
#25138=DIRECTION('ref_axis',(-0.707106781186548,0.707106781186547,3.74194010293243E-33));
#25139=DIRECTION('',(-1.00027490415113E-12,0.,-1.));
#25140=DIRECTION('',(0.678598344545735,-0.678598344545736,-0.281084637715359));
#25141=DIRECTION('',(1.00027490415113E-12,0.,1.));
#25142=DIRECTION('',(0.678598344545735,-0.678598344545735,0.281084637715361));
#25143=DIRECTION('center_axis',(-0.500000000000001,-0.707106781186547,0.500000000000001));
#25144=DIRECTION('ref_axis',(-0.816496580927725,0.577350269189627,2.5034978194734E-16));
#25145=DIRECTION('',(-0.707106781186548,0.,-0.707106781186547));
#25146=DIRECTION('',(0.281084637715357,-0.678598344545735,-0.678598344545737));
#25147=DIRECTION('',(0.707106781186548,0.,0.707106781186547));
#25148=DIRECTION('center_axis',(9.71932950752329E-17,-0.707106781186548,
0.707106781186547));
#25149=DIRECTION('ref_axis',(-1.,-1.37452076067124E-16,2.07747144876332E-31));
#25150=DIRECTION('',(-1.,0.,1.00013745207507E-12));
#25151=DIRECTION('',(-0.281084637715359,-0.678598344545735,-0.678598344545736));
#25152=DIRECTION('',(1.,0.,-1.00013745207507E-12));
#25153=DIRECTION('center_axis',(0.5,-0.707106781186547,0.5));
#25154=DIRECTION('ref_axis',(1.18404905982997E-16,-0.577350269189626,-0.816496580927726));
#25155=DIRECTION('',(0.707106781186547,0.,-0.707106781186548));
#25156=DIRECTION('',(-0.707106781186547,0.,0.707106781186548));
#25157=DIRECTION('',(-0.678598344545736,-0.678598344545735,-0.281084637715358));
#25158=DIRECTION('center_axis',(0.707106781186547,-0.707106781186548,-9.71932950752329E-17));
#25159=DIRECTION('ref_axis',(-2.09730162168143E-31,1.37452076067124E-16,
-1.));
#25160=DIRECTION('',(-1.00013745207507E-12,0.,-1.));
#25161=DIRECTION('',(1.00013745207507E-12,0.,1.));
#25162=DIRECTION('',(-0.678598344545735,-0.678598344545735,0.28108463771536));
#25163=DIRECTION('center_axis',(0.5,-0.707106781186548,-0.5));
#25164=DIRECTION('ref_axis',(-1.2120878851009E-16,0.577350269189625,-0.816496580927726));
#25165=DIRECTION('',(-0.707106781186548,0.,-0.707106781186548));
#25166=DIRECTION('',(0.707106781186548,0.,0.707106781186548));
#25167=DIRECTION('',(-0.281084637715359,-0.678598344545735,0.678598344545736));
#25168=DIRECTION('center_axis',(0.,-0.707106781186548,-0.707106781186547));
#25169=DIRECTION('ref_axis',(0.,0.707106781186547,-0.707106781186548));
#25170=DIRECTION('',(-1.,0.,0.));
#25171=DIRECTION('',(1.,0.,0.));
#25172=DIRECTION('',(0.281084637715361,-0.678598344545735,0.678598344545735));
#25173=DIRECTION('center_axis',(-0.5,-0.707106781186548,-0.5));
#25174=DIRECTION('ref_axis',(1.2120878851009E-16,0.577350269189625,-0.816496580927726));
#25175=DIRECTION('',(-0.707106781186548,0.,0.707106781186548));
#25176=DIRECTION('',(0.707106781186548,0.,-0.707106781186548));
#25177=DIRECTION('center_axis',(-0.707106781186548,0.,0.707106781186548));
#25178=DIRECTION('ref_axis',(0.,1.,0.));
#25179=DIRECTION('',(0.,1.,0.));
#25180=DIRECTION('',(0.,1.,0.));
#25181=DIRECTION('center_axis',(0.,0.,1.));
#25182=DIRECTION('ref_axis',(1.,0.,0.));
#25183=DIRECTION('',(0.,1.,0.));
#25184=DIRECTION('center_axis',(0.707106781186548,0.,0.707106781186548));
#25185=DIRECTION('ref_axis',(0.,-1.,0.));
#25186=DIRECTION('',(0.,1.,0.));
#25187=DIRECTION('center_axis',(1.,0.,-2.74904152134249E-16));
#25188=DIRECTION('ref_axis',(0.,1.,0.));
#25189=DIRECTION('',(0.,1.,0.));
#25190=DIRECTION('center_axis',(0.,-1.,0.));
#25191=DIRECTION('ref_axis',(0.,0.,-1.));
#25192=DIRECTION('center_axis',(0.,-1.,0.));
#25193=DIRECTION('ref_axis',(-1.,0.,0.));
#25194=DIRECTION('center_axis',(0.700909264299845,0.713250449154187,0.));
#25195=DIRECTION('ref_axis',(0.,0.,-1.));
#25196=DIRECTION('',(0.,0.,-1.));
#25197=DIRECTION('center_axis',(0.,-1.,0.));
#25198=DIRECTION('ref_axis',(-1.,0.,0.));
#25199=DIRECTION('center_axis',(0.,1.,0.));
#25200=DIRECTION('ref_axis',(-1.,0.,0.));
#25201=DIRECTION('',(-0.707106781186547,0.707106781186548,-8.65956056235492E-17));
#25202=DIRECTION('center_axis',(0.,-1.,0.));
#25203=DIRECTION('ref_axis',(-1.,0.,0.));
#25204=DIRECTION('center_axis',(0.,1.,0.));
#25205=DIRECTION('ref_axis',(-1.,0.,0.));
#25206=DIRECTION('center_axis',(0.,1.,0.));
#25207=DIRECTION('ref_axis',(1.,0.,0.));
#25208=DIRECTION('center_axis',(0.,1.,0.));
#25209=DIRECTION('ref_axis',(-1.,0.,0.));
#25210=DIRECTION('center_axis',(0.,1.,0.));
#25211=DIRECTION('ref_axis',(1.,0.,0.));
#25212=DIRECTION('',(0.,-1.,0.));
#25213=DIRECTION('center_axis',(0.,1.,0.));
#25214=DIRECTION('ref_axis',(-1.,0.,0.));
#25215=DIRECTION('center_axis',(0.,-1.,0.));
#25216=DIRECTION('ref_axis',(-1.,0.,0.));
#25217=DIRECTION('',(0.707106781186545,0.70710678118655,-8.6595605623549E-17));
#25218=DIRECTION('center_axis',(0.,-1.,0.));
#25219=DIRECTION('ref_axis',(-1.,0.,0.));
#25220=DIRECTION('center_axis',(0.,1.,0.));
#25221=DIRECTION('ref_axis',(1.,0.,0.));
#25222=DIRECTION('center_axis',(0.,1.,0.));
#25223=DIRECTION('ref_axis',(1.,0.,0.));
#25224=DIRECTION('',(0.,1.,0.));
#25225=DIRECTION('center_axis',(0.,-1.,0.));
#25226=DIRECTION('ref_axis',(1.,0.,0.));
#25227=DIRECTION('',(-0.707106781186544,-0.707106781186551,-8.65956056235488E-17));
#25228=DIRECTION('center_axis',(0.,-1.,0.));
#25229=DIRECTION('ref_axis',(1.,0.,0.));
#25230=DIRECTION('center_axis',(0.,-1.,0.));
#25231=DIRECTION('ref_axis',(0.,0.,-1.));
#25232=DIRECTION('center_axis',(0.,1.,0.));
#25233=DIRECTION('ref_axis',(1.,0.,0.));
#25234=DIRECTION('center_axis',(0.,1.,0.));
#25235=DIRECTION('ref_axis',(-1.,0.,0.));
#25236=DIRECTION('center_axis',(0.,-1.,0.));
#25237=DIRECTION('ref_axis',(-1.,0.,0.));
#25238=DIRECTION('',(-0.707106781186546,-0.707106781186549,8.65956056235491E-17));
#25239=DIRECTION('center_axis',(0.,1.,0.));
#25240=DIRECTION('ref_axis',(-1.,0.,0.));
#25241=DIRECTION('center_axis',(0.,-1.,0.));
#25242=DIRECTION('ref_axis',(0.,0.,-1.));
#25243=DIRECTION('center_axis',(0.,-1.,0.));
#25244=DIRECTION('ref_axis',(-1.,0.,0.));
#25245=DIRECTION('center_axis',(0.,1.,0.));
#25246=DIRECTION('ref_axis',(-1.,0.,0.));
#25247=DIRECTION('',(0.,-1.,0.));
#25248=DIRECTION('center_axis',(0.,-1.,0.));
#25249=DIRECTION('ref_axis',(-1.,0.,0.));
#25250=DIRECTION('center_axis',(0.,1.,0.));
#25251=DIRECTION('ref_axis',(-1.,0.,0.));
#25252=DIRECTION('',(0.242535625036333,-0.970142500145332,2.97020476879948E-17));
#25253=DIRECTION('center_axis',(0.,1.,0.));
#25254=DIRECTION('ref_axis',(-1.,0.,0.));
#25255=DIRECTION('center_axis',(0.,1.,0.));
#25256=DIRECTION('ref_axis',(1.,0.,0.));
#25257=DIRECTION('',(0.,1.,0.));
#25258=DIRECTION('center_axis',(0.,1.,0.));
#25259=DIRECTION('ref_axis',(1.,0.,0.));
#25260=DIRECTION('center_axis',(0.,1.,0.));
#25261=DIRECTION('ref_axis',(1.,0.,0.));
#25262=DIRECTION('',(0.,1.,0.));
#25263=DIRECTION('center_axis',(0.,1.,0.));
#25264=DIRECTION('ref_axis',(1.,0.,0.));
#25265=DIRECTION('',(0.,1.,0.));
#25266=DIRECTION('center_axis',(0.,1.,0.));
#25267=DIRECTION('ref_axis',(1.,0.,0.));
#25268=DIRECTION('',(0.,1.,0.));
#25269=DIRECTION('center_axis',(0.,1.,0.));
#25270=DIRECTION('ref_axis',(1.,0.,0.));
#25271=DIRECTION('',(0.,1.,0.));
#25272=DIRECTION('center_axis',(0.,1.,0.));
#25273=DIRECTION('ref_axis',(1.,0.,0.));
#25274=DIRECTION('center_axis',(0.,1.,0.));
#25275=DIRECTION('ref_axis',(1.,0.,0.));
#25276=DIRECTION('',(0.,1.,0.));
#25277=DIRECTION('center_axis',(0.,-1.,0.));
#25278=DIRECTION('ref_axis',(0.,0.,-1.));
#25279=DIRECTION('center_axis',(-1.,0.,1.37452076067125E-16));
#25280=DIRECTION('ref_axis',(0.,1.,0.));
#25281=DIRECTION('',(0.,1.,0.));
#25282=DIRECTION('center_axis',(-0.707106781186548,0.,-0.707106781186547));
#25283=DIRECTION('ref_axis',(-0.707106781186547,0.,0.707106781186548));
#25284=DIRECTION('',(0.,1.,0.));
#25285=DIRECTION('center_axis',(-1.37452076067125E-16,0.,-1.));
#25286=DIRECTION('ref_axis',(-1.,0.,1.37452076067125E-16));
#25287=DIRECTION('',(0.,1.,0.));
#25288=DIRECTION('center_axis',(0.707106781186547,0.,-0.707106781186548));
#25289=DIRECTION('ref_axis',(0.,-1.,0.));
#25290=DIRECTION('center_axis',(0.999847695156391,0.0174524064372833,0.));
#25291=DIRECTION('ref_axis',(0.,0.,-1.));
#31308=CARTESIAN_POINT('',(0.,0.,0.));
#31309=CARTESIAN_POINT('Origin',(0.0129631448730721,-0.024,0.0191500000000096));
#31310=CARTESIAN_POINT('',(0.014084281726958,-0.008,0.0208062162162298));
#31311=CARTESIAN_POINT('',(0.0131664441683726,-0.00800000000001,0.0211396405194357));
#31312=CARTESIAN_POINT('Origin',(0.0129631448730721,-0.008,0.0191500000000096));
#31313=CARTESIAN_POINT('',(0.014084281726958,-5.52435218316827E-5,0.0208062162162298));
#31314=CARTESIAN_POINT('',(0.014084281726958,-0.024,0.0208062162162298));
#31315=CARTESIAN_POINT('',(0.0137123694638326,-0.0002499619237991,0.0210043631016193));
#31316=CARTESIAN_POINT('Origin',(0.0129631448730721,0.00157231562097569,
0.0191500000000096));
#31317=CARTESIAN_POINT('Origin',(0.0129631448730721,0.105986429016355,0.0191500000000096));
#31318=CARTESIAN_POINT('Origin',(-1.00275343584144E-14,-0.024,9.9475983006414E-15));
#31319=CARTESIAN_POINT('',(0.020806216216238,-0.008,0.0140842817269634));
#31320=CARTESIAN_POINT('Origin',(-1.00275343584144E-14,-0.008,9.9475983006414E-15));
#31321=CARTESIAN_POINT('',(0.020806216216238,-5.52435218397962E-5,0.0140842817269634));
#31322=CARTESIAN_POINT('',(0.020806216216238,-0.024,0.0140842817269634));
#31323=CARTESIAN_POINT('',(0.02075000000001,0.,0.014166973035935));
#31324=CARTESIAN_POINT('Origin',(-1.00275343584144E-14,0.0203909682096601,
9.9475983006414E-15));
#31325=CARTESIAN_POINT('',(0.0141669730359443,0.,0.02075000000001));
#31326=CARTESIAN_POINT('Origin',(-1.00275343584144E-14,0.,9.9475983006414E-15));
#31327=CARTESIAN_POINT('Origin',(-1.00275343584144E-14,0.0203909682096408,
9.9475983006414E-15));
#31328=CARTESIAN_POINT('Origin',(-0.0191500000000098,-0.024,0.0129631448730722));
#31329=CARTESIAN_POINT('',(-0.0208062162162391,-0.008,0.0140842817269642));
#31330=CARTESIAN_POINT('',(-0.0211396405194357,-0.00800000000001,0.013166444168483));
#31331=CARTESIAN_POINT('Origin',(-0.0191500000000098,-0.008,0.0129631448730722));
#31332=CARTESIAN_POINT('',(-0.0208062162162391,-5.52435218408842E-5,0.0140842817269642));
#31333=CARTESIAN_POINT('',(-0.0208062162162391,-0.024,0.0140842817269642));
#31334=CARTESIAN_POINT('',(-0.0210043631016193,-0.0002499619237991,0.0137123694638626));
#31335=CARTESIAN_POINT('Origin',(-0.0191500000000098,0.00157231562097551,
0.0129631448730722));
#31336=CARTESIAN_POINT('Origin',(-0.0191500000000098,0.105986429016344,
0.0129631448730722));
#31337=CARTESIAN_POINT('Origin',(-1.00275343584144E-14,-0.024,9.9475983006414E-15));
#31338=CARTESIAN_POINT('',(-0.0140842817269636,-0.008,0.0208062162162381));
#31339=CARTESIAN_POINT('Origin',(-1.00275343584144E-14,-0.008,9.9475983006414E-15));
#31340=CARTESIAN_POINT('',(-0.0140842817269636,-5.52435218398184E-5,0.0208062162162381));
#31341=CARTESIAN_POINT('',(-0.0140842817269636,-0.024,0.0208062162162381));
#31342=CARTESIAN_POINT('',(-0.0141669730359351,0.,0.02075000000001));
#31343=CARTESIAN_POINT('Origin',(-1.00275343584144E-14,0.0203909682096408,
9.9475983006414E-15));
#31344=CARTESIAN_POINT('',(-0.02075000000001,0.,0.0141669730359352));
#31345=CARTESIAN_POINT('Origin',(-1.00275343584144E-14,0.,9.9475983006414E-15));
#31346=CARTESIAN_POINT('Origin',(-1.00275343584144E-14,0.0203909682096408,
9.9475983006414E-15));
#31347=CARTESIAN_POINT('Origin',(-0.0129631448730721,-0.024,-0.0191500000000097));
#31348=CARTESIAN_POINT('',(-0.014084281726955,-0.008,-0.0208062162162255));
#31349=CARTESIAN_POINT('',(-0.0131664441683213,-0.00800000000001,-0.0211396405194357));
#31350=CARTESIAN_POINT('Origin',(-0.0129631448730721,-0.008,-0.0191500000000097));
#31351=CARTESIAN_POINT('',(-0.014084281726955,-5.52435218274594E-5,-0.0208062162162255));
#31352=CARTESIAN_POINT('',(-0.014084281726955,-0.024,-0.0208062162162255));
#31353=CARTESIAN_POINT('',(-0.0137123694638187,-0.0002499619237991,-0.0210043631016193));
#31354=CARTESIAN_POINT('Origin',(-0.0129631448730721,0.00157231562097559,
-0.0191500000000097));
#31355=CARTESIAN_POINT('Origin',(-0.0129631448730721,0.105986429016349,
-0.0191500000000097));
#31356=CARTESIAN_POINT('Origin',(-1.00275343584144E-14,-0.024,9.9475983006414E-15));
#31357=CARTESIAN_POINT('',(-0.0208062162162194,-0.008,-0.0140842817269509));
#31358=CARTESIAN_POINT('Origin',(-1.00275343584144E-14,-0.008,9.9475983006414E-15));
#31359=CARTESIAN_POINT('',(-0.0208062162162194,-5.52435218215264E-5,-0.0140842817269509));
#31360=CARTESIAN_POINT('',(-0.0208062162162194,-0.024,-0.0140842817269509));
#31361=CARTESIAN_POINT('',(-0.02075000000001,0.,-0.0141669730359175));
#31362=CARTESIAN_POINT('Origin',(-1.00275343584144E-14,0.0203909682096408,
9.9475983006414E-15));
#31363=CARTESIAN_POINT('',(-0.0141669730359082,0.,-0.02075000000001));
#31364=CARTESIAN_POINT('Origin',(-1.00275343584144E-14,0.,9.9475983006414E-15));
#31365=CARTESIAN_POINT('Origin',(-1.00275343584144E-14,0.0203909682096604,
9.9475983006414E-15));
#31366=CARTESIAN_POINT('Origin',(0.01915000000001,-0.024,-0.0129631448730722));
#31367=CARTESIAN_POINT('',(0.0208062162162161,-0.008,-0.0140842817269487));
#31368=CARTESIAN_POINT('',(0.0211396405194357,-0.00800000000001,-0.0131664441682106));
#31369=CARTESIAN_POINT('Origin',(0.01915000000001,-0.008,-0.0129631448730722));
#31370=CARTESIAN_POINT('',(0.0208062162162161,-5.52435218182845E-5,-0.0140842817269487));
#31371=CARTESIAN_POINT('',(0.0208062162162161,-0.024,-0.0140842817269487));
#31372=CARTESIAN_POINT('',(0.0210043631016193,-0.0002499619237991,-0.0137123694637886));
#31373=CARTESIAN_POINT('Origin',(0.01915000000001,0.00157231562097526,-0.0129631448730722));
#31374=CARTESIAN_POINT('Origin',(0.01915000000001,0.105986429016332,-0.0129631448730722));
#31375=CARTESIAN_POINT('Origin',(-1.00275343584144E-14,-0.024,9.9475983006414E-15));
#31376=CARTESIAN_POINT('',(0.0140842817269635,-0.008,-0.0208062162162381));
#31377=CARTESIAN_POINT('Origin',(-1.00275343584144E-14,-0.008,9.9475983006414E-15));
#31378=CARTESIAN_POINT('',(0.0140842817269635,-5.52435218398539E-5,-0.0208062162162381));
#31379=CARTESIAN_POINT('',(0.0140842817269635,-0.024,-0.0208062162162381));
#31380=CARTESIAN_POINT('',(0.0141669730358881,0.,-0.02075000000001));
#31381=CARTESIAN_POINT('Origin',(-1.00275343584144E-14,0.0203909682096604,
9.9475983006414E-15));
#31382=CARTESIAN_POINT('',(0.02075000000001,0.,-0.0141669730358881));
#31383=CARTESIAN_POINT('Origin',(-1.00275343584144E-14,0.,9.9475983006414E-15));
#31384=CARTESIAN_POINT('Origin',(-1.00275343584144E-14,0.0203909682096601,
9.9475983006414E-15));
#31385=CARTESIAN_POINT('Origin',(0.01915000000001,-0.024,0.0129631448730722));
#31386=CARTESIAN_POINT('',(0.0211396405194357,-0.00800000000001,0.0131664441682491));
#31387=CARTESIAN_POINT('Origin',(0.01915000000001,-0.008,0.0129631448730722));
#31388=CARTESIAN_POINT('',(0.0210043631016193,-0.0002499619237991,0.0137123694637991));
#31389=CARTESIAN_POINT('Origin',(0.01915000000001,0.105986429016333,0.0129631448730722));
#31390=CARTESIAN_POINT('Origin',(0.01915000000001,0.00157231562097527,0.0129631448730722));
#31391=CARTESIAN_POINT('Origin',(-0.0129631448730724,-0.024,0.0191500000000103));
#31392=CARTESIAN_POINT('',(-0.0131664441682495,-0.00800000000001,0.0211396405194357));
#31393=CARTESIAN_POINT('Origin',(-0.0129631448730724,-0.008,0.0191500000000103));
#31394=CARTESIAN_POINT('',(-0.0137123694637993,-0.0002499619237991,0.0210043631016193));
#31395=CARTESIAN_POINT('Origin',(-0.0129631448730724,0.105986429016316,
0.0191500000000103));
#31396=CARTESIAN_POINT('Origin',(-0.0129631448730724,0.00157231562097503,
0.0191500000000103));
#31397=CARTESIAN_POINT('Origin',(-0.01915000000001,-0.024,-0.0129631448730723));
#31398=CARTESIAN_POINT('',(-0.0211396405194357,-0.00800000000001,-0.0131664441682492));
#31399=CARTESIAN_POINT('Origin',(-0.01915000000001,-0.008,-0.0129631448730723));
#31400=CARTESIAN_POINT('',(-0.0210043631016193,-0.0002499619237991,-0.0137123694637992));
#31401=CARTESIAN_POINT('Origin',(-0.01915000000001,0.105986429016332,-0.0129631448730723));
#31402=CARTESIAN_POINT('Origin',(-0.01915000000001,0.00157231562097529,
-0.0129631448730723));
#31403=CARTESIAN_POINT('Origin',(0.012963144873072,-0.024,-0.0191500000000096));
#31404=CARTESIAN_POINT('',(0.0131664441684711,-0.00800000000001,-0.0211396405194357));
#31405=CARTESIAN_POINT('Origin',(0.012963144873072,-0.008,-0.0191500000000096));
#31406=CARTESIAN_POINT('',(0.0137123694638593,-0.0002499619237991,-0.0210043631016193));
#31407=CARTESIAN_POINT('Origin',(0.012963144873072,0.105986429016355,-0.0191500000000096));
#31408=CARTESIAN_POINT('Origin',(0.012963144873072,0.00157231562097569,
-0.0191500000000096));
#31409=CARTESIAN_POINT('Origin',(-0.016,0.,0.021));
#31410=CARTESIAN_POINT('',(-0.00800000000001,-0.000249961923799098,0.0210043631016193));
#31411=CARTESIAN_POINT('',(-0.01600000000001,-0.00800000000001,0.0211396405194357));
#31412=CARTESIAN_POINT('Origin',(-0.008,-0.000124980961894549,0.0208771815508047));
#31413=CARTESIAN_POINT('',(-0.00800000000001,0.,0.02075000000001));
#31414=CARTESIAN_POINT('Origin',(-0.021,0.,-0.016));
#31415=CARTESIAN_POINT('',(-0.0210043631016193,-0.000249961923799098,-0.00800000000001));
#31416=CARTESIAN_POINT('',(-0.0211396405194357,-0.00800000000001,-0.01600000000001));
#31417=CARTESIAN_POINT('Origin',(-0.0208771815508047,-0.000124980961894549,
-0.008));
#31418=CARTESIAN_POINT('',(-0.02075000000001,0.,-0.00800000000001));
#31419=CARTESIAN_POINT('Origin',(0.016,0.,-0.021));
#31420=CARTESIAN_POINT('',(0.00800000000001,-0.000249961923799098,-0.0210043631016193));
#31421=CARTESIAN_POINT('',(0.01600000000001,-0.00800000000001,-0.0211396405194357));
#31422=CARTESIAN_POINT('Origin',(2.22044604925031E-18,-0.008,0.));
#31423=CARTESIAN_POINT('',(0.0211396405194357,-0.00800000000001,0.01600000000001));
#31424=CARTESIAN_POINT('',(0.00807716446627536,-0.008,0.0195));
#31425=CARTESIAN_POINT('',(0.0195,-0.008,0.00807716446627536));
#31426=CARTESIAN_POINT('',(0.0109328733497165,-0.00800000000001,0.0166442911165789));
#31427=CARTESIAN_POINT('',(0.0195,-0.008,-0.00807716446627536));
#31428=CARTESIAN_POINT('',(0.01950000000001,-0.00800000000001,0.00403858223314768));
#31429=CARTESIAN_POINT('',(0.00807716446627536,-0.008,-0.0195));
#31430=CARTESIAN_POINT('',(0.0166442911165789,-0.00800000000001,-0.0109328733497165));
#31431=CARTESIAN_POINT('',(-0.00807716446627536,-0.008,-0.0195));
#31432=CARTESIAN_POINT('',(0.00403858223314768,-0.00800000000001,-0.01950000000001));
#31433=CARTESIAN_POINT('',(-0.0195,-0.008,-0.00807716446627536));
#31434=CARTESIAN_POINT('',(-0.0109328733497165,-0.00800000000001,-0.0166442911165788));
#31435=CARTESIAN_POINT('',(-0.0195,-0.008,0.00807716446627536));
#31436=CARTESIAN_POINT('',(-0.01950000000001,-0.00800000000001,-0.00403858223314768));
#31437=CARTESIAN_POINT('',(-0.00807716446627536,-0.008,0.0195));
#31438=CARTESIAN_POINT('',(-0.0166442911165788,-0.00800000000001,0.0109328733497165));
#31439=CARTESIAN_POINT('',(-0.00403858223314768,-0.00800000000001,0.01950000000001));
#31440=CARTESIAN_POINT('',(-0.0167295,-0.00800000000001,0.0155));
#31441=CARTESIAN_POINT('Origin',(-0.01550000000001,-0.00800000000001,0.01550000000001));
#31442=CARTESIAN_POINT('',(0.0142705,-0.00800000000001,-0.0155));
#31443=CARTESIAN_POINT('Origin',(0.01550000000001,-0.00800000000001,-0.01550000000001));
#31444=CARTESIAN_POINT('',(-0.0167295,-0.00800000000001,-0.0155));
#31445=CARTESIAN_POINT('Origin',(-0.01550000000001,-0.00800000000001,-0.01550000000001));
#31446=CARTESIAN_POINT('',(0.0142705,-0.00800000000001,0.0155));
#31447=CARTESIAN_POINT('Origin',(0.01550000000001,-0.00800000000001,0.01550000000001));
#31448=CARTESIAN_POINT('Origin',(0.008,-0.000124980961894549,-0.0208771815508047));
#31449=CARTESIAN_POINT('',(0.00800000000001,0.,-0.02075000000001));
#31450=CARTESIAN_POINT('Origin',(2.22044604925031E-18,0.,0.));
#31451=CARTESIAN_POINT('',(0.02075000000001,0.,0.00800000000001));
#31452=CARTESIAN_POINT('',(0.0142705,0.,0.0155));
#31453=CARTESIAN_POINT('Origin',(0.01550000000001,0.,0.01550000000001));
#31454=CARTESIAN_POINT('',(-0.0167295,0.,-0.0155));
#31455=CARTESIAN_POINT('Origin',(-0.01550000000001,0.,-0.01550000000001));
#31456=CARTESIAN_POINT('',(0.0142705,0.,-0.0155));
#31457=CARTESIAN_POINT('Origin',(0.01550000000001,0.,-0.01550000000001));
#31458=CARTESIAN_POINT('',(-0.0167295,0.,0.0155));
#31459=CARTESIAN_POINT('Origin',(-0.01550000000001,0.,0.01550000000001));
#31460=CARTESIAN_POINT('',(-0.0109,0.,1.33486501107061E-18));
#31461=CARTESIAN_POINT('Origin',(0.,0.,0.));
#31462=CARTESIAN_POINT('Origin',(0.019,-0.0025,0.00403858223313768));
#31463=CARTESIAN_POINT('',(0.0185,-0.002,0.00766295090390226));
#31464=CARTESIAN_POINT('',(0.0185,-0.002,-0.00766295090390227));
#31465=CARTESIAN_POINT('',(0.01850000000001,-0.00200000000001,0.00403858223314768));
#31466=CARTESIAN_POINT('',(0.0195,-0.003,-0.00807716446627536));
#31467=CARTESIAN_POINT('',(0.01850000000001,-0.00200000000001,-0.00766295090391227));
#31468=CARTESIAN_POINT('',(0.0195,-0.003,0.00807716446627536));
#31469=CARTESIAN_POINT('',(0.01950000000001,-0.00300000000001,0.00403858223314768));
#31470=CARTESIAN_POINT('',(0.01850000000001,-0.00200000000001,0.00766295090391226));
#31471=CARTESIAN_POINT('Origin',(0.0162907377259756,-0.0025,-0.0105793199591133));
#31472=CARTESIAN_POINT('',(0.00766295090390227,-0.002,-0.0185));
#31473=CARTESIAN_POINT('',(0.0159371843353923,-0.00200000000001,-0.01022576656853));
#31474=CARTESIAN_POINT('',(0.00807716446627536,-0.003,-0.0195));
#31475=CARTESIAN_POINT('',(0.00766295090391227,-0.00200000000001,-0.01850000000001));
#31476=CARTESIAN_POINT('',(0.0166442911165789,-0.00300000000001,-0.0109328733497165));
#31477=CARTESIAN_POINT('Origin',(0.00403858223313768,-0.0025,-0.019));
#31478=CARTESIAN_POINT('',(-0.00766295090390227,-0.002,-0.0185));
#31479=CARTESIAN_POINT('',(0.00403858223314768,-0.00200000000001,-0.01850000000001));
#31480=CARTESIAN_POINT('',(-0.00807716446627536,-0.003,-0.0195));
#31481=CARTESIAN_POINT('',(-0.00766295090391227,-0.00200000000001,-0.01850000000001));
#31482=CARTESIAN_POINT('',(0.00403858223314768,-0.00300000000001,-0.01950000000001));
#31483=CARTESIAN_POINT('Origin',(-0.0105793199591133,-0.0025,-0.0162907377259756));
#31484=CARTESIAN_POINT('',(-0.0195,-0.003,-0.00807716446627536));
#31485=CARTESIAN_POINT('',(-0.0109328733497165,-0.00300000000001,-0.0166442911165788));
#31486=CARTESIAN_POINT('',(-0.0185,-0.002,-0.00766295090390226));
#31487=CARTESIAN_POINT('',(-0.01022576656853,-0.00200000000001,-0.0159371843353923));
#31488=CARTESIAN_POINT('',(-0.01850000000001,-0.00200000000001,-0.00766295090391226));
#31489=CARTESIAN_POINT('Origin',(-0.019,-0.0025,-0.00403858223313768));
#31490=CARTESIAN_POINT('',(-0.0195,-0.003,0.00807716446627536));
#31491=CARTESIAN_POINT('',(-0.01950000000001,-0.00300000000001,-0.00403858223314768));
#31492=CARTESIAN_POINT('',(-0.0185,-0.002,0.00766295090390227));
#31493=CARTESIAN_POINT('',(-0.01850000000001,-0.00200000000001,-0.00403858223314768));
#31494=CARTESIAN_POINT('',(-0.01850000000001,-0.00200000000001,0.00766295090391227));
#31495=CARTESIAN_POINT('Origin',(-0.0162907377259756,-0.0025,0.0105793199591132));
#31496=CARTESIAN_POINT('',(-0.00807716446627536,-0.003,0.0195));
#31497=CARTESIAN_POINT('',(-0.0166442911165789,-0.00300000000001,0.0109328733497165));
#31498=CARTESIAN_POINT('',(-0.00766295090390226,-0.002,0.0185));
#31499=CARTESIAN_POINT('',(-0.0159371843353923,-0.00200000000001,0.01022576656853));
#31500=CARTESIAN_POINT('',(-0.00766295090391226,-0.00200000000001,0.01850000000001));
#31501=CARTESIAN_POINT('Origin',(-0.00403858223313768,-0.0025,0.019));
#31502=CARTESIAN_POINT('',(0.00807716446627536,-0.003,0.0195));
#31503=CARTESIAN_POINT('',(-0.00403858223314768,-0.00300000000001,0.01950000000001));
#31504=CARTESIAN_POINT('',(0.00766295090390227,-0.002,0.0185));
#31505=CARTESIAN_POINT('',(-0.00403858223314768,-0.00200000000001,0.01850000000001));
#31506=CARTESIAN_POINT('',(0.00766295090391227,-0.00200000000001,0.01850000000001));
#31507=CARTESIAN_POINT('Origin',(0.0105793199591133,-0.0025,0.0162907377259756));
#31508=CARTESIAN_POINT('',(0.0109328733497165,-0.00300000000001,0.0166442911165789));
#31509=CARTESIAN_POINT('',(0.01022576656853,-0.00200000000001,0.0159371843353923));
#31510=CARTESIAN_POINT('Origin',(-0.0195,-0.008,0.00807716446627536));
#31511=CARTESIAN_POINT('',(-0.00807716446628536,-0.00800000000001,0.01950000000001));
#31512=CARTESIAN_POINT('',(-0.01950000000001,-0.00800000000001,0.00807716446628536));
#31513=CARTESIAN_POINT('Origin',(-0.00807716446627536,-0.008,0.0195));
#31514=CARTESIAN_POINT('',(0.00807716446628536,-0.00800000000001,0.01950000000001));
#31515=CARTESIAN_POINT('Origin',(0.00807716446627536,-0.008,0.0195));
#31516=CARTESIAN_POINT('',(0.01950000000001,-0.00800000000001,0.00807716446628536));
#31517=CARTESIAN_POINT('Origin',(0.0195,-0.008,0.00807716446627536));
#31518=CARTESIAN_POINT('',(0.01950000000001,-0.00800000000001,-0.00807716446628536));
#31519=CARTESIAN_POINT('Origin',(3.33066907387547E-18,-0.002,-1.11022302462516E-18));
#31520=CARTESIAN_POINT('',(0.013,-0.00200000000001,-1.59204083889156E-18));
#31521=CARTESIAN_POINT('Origin',(0.,-0.00200000000001,0.));
#31522=CARTESIAN_POINT('Origin',(0.0208771815508047,-0.000124980961894549,
0.008));
#31523=CARTESIAN_POINT('',(0.0210043631016193,-0.000249961923799098,0.00800000000001));
#31524=CARTESIAN_POINT('Origin',(0.,0.001875,0.));
#31525=CARTESIAN_POINT('',(-0.01090000000001,0.00175000000001,0.));
#31526=CARTESIAN_POINT('',(0.0109,0.00175,1.33486501107062E-18));
#31527=CARTESIAN_POINT('Origin',(0.,0.00175000000001,0.));
#31528=CARTESIAN_POINT('',(0.01065,0.002,1.30424884109193E-18));
#31529=CARTESIAN_POINT('',(0.010775,0.001875,1.31955692608127E-18));
#31530=CARTESIAN_POINT('Origin',(0.,0.00200000000001,0.));
#31531=CARTESIAN_POINT('Origin',(0.,0.00175000000001,0.));
#31532=CARTESIAN_POINT('Origin',(0.,0.002,0.));
#31533=CARTESIAN_POINT('',(0.00475000000001,0.00200000000001,-5.81707229596217E-19));
#31534=CARTESIAN_POINT('Origin',(0.,0.00200000000001,0.));
#31535=CARTESIAN_POINT('Origin',(0.,0.,0.));
#31536=CARTESIAN_POINT('',(-0.0109,0.,1.33486501107061E-18));
#31537=CARTESIAN_POINT('Origin',(0.,0.001875,0.));
#31538=CARTESIAN_POINT('',(-0.00450000000001,0.00175000000001,0.));
#31539=CARTESIAN_POINT('',(0.00450000000001,0.00175000000001,-5.51091059617534E-19));
#31540=CARTESIAN_POINT('Origin',(0.,0.00175000000001,0.));
#31541=CARTESIAN_POINT('',(0.004625,0.001875,-5.66399144605651E-19));
#31542=CARTESIAN_POINT('Origin',(0.,0.00175000000001,0.));
#31543=CARTESIAN_POINT('Origin',(0.,-0.0587953551706409,0.));
#31544=CARTESIAN_POINT('',(-0.0045,0.000250000000010004,5.51091059616309E-19));
#31545=CARTESIAN_POINT('Origin',(0.,0.000250000000010004,0.));
#31546=CARTESIAN_POINT('',(-0.0045,-0.0587953551706409,5.51091059616309E-19));
#31547=CARTESIAN_POINT('Origin',(0.,0.000125000000000002,0.));
#31548=CARTESIAN_POINT('',(-0.00475,5.72458747072346E-19,-5.81707229594993E-19));
#31549=CARTESIAN_POINT('',(-0.004625,0.000125000000000002,-5.66399144605651E-19));
#31550=CARTESIAN_POINT('Origin',(0.,1.00005551115123E-14,0.));
#31551=CARTESIAN_POINT('Origin',(0.,5.55111512312578E-19,0.));
#31552=CARTESIAN_POINT('',(-0.006,1.00006114500673E-14,7.34788079488412E-19));
#31553=CARTESIAN_POINT('Origin',(0.,1.00005551115123E-14,0.));
#31554=CARTESIAN_POINT('Origin',(0.,-0.008875,0.));
#31555=CARTESIAN_POINT('',(0.013,-0.00875,-1.59204083889156E-18));
#31556=CARTESIAN_POINT('Origin',(0.,-0.00875000000001,0.));
#31557=CARTESIAN_POINT('',(0.01275,-0.009,-1.56142466891288E-18));
#31558=CARTESIAN_POINT('',(0.012875,-0.008875,-1.57673275390222E-18));
#31559=CARTESIAN_POINT('Origin',(0.,-0.00900000000001,0.));
#31560=CARTESIAN_POINT('Origin',(0.,-0.009,0.));
#31561=CARTESIAN_POINT('',(0.00825000000000294,-0.00900000000001176,1.01033360929693E-18));
#31562=CARTESIAN_POINT('Origin',(0.,-0.00900000000001,0.));
#31563=CARTESIAN_POINT('Origin',(0.,-0.008,0.));
#31564=CARTESIAN_POINT('',(0.013,-0.008,-1.59204083889156E-18));
#31565=CARTESIAN_POINT('Origin',(0.,-0.0085,0.));
#31566=CARTESIAN_POINT('',(-0.00800000000001,-0.00800000000001,0.));
#31567=CARTESIAN_POINT('',(0.00800000000000294,-0.00800000000001177,9.79717439318243E-19));
#31568=CARTESIAN_POINT('Origin',(0.,-0.00800000000001,0.));
#31569=CARTESIAN_POINT('',(0.008125,-0.0085,9.95025524307224E-19));
#31570=CARTESIAN_POINT('Origin',(0.,-0.00800000000001,0.));
#31571=CARTESIAN_POINT('Origin',(0.,-0.009,0.));
#31572=CARTESIAN_POINT('',(-0.008,-0.000750000000010002,9.79717439317883E-19));
#31573=CARTESIAN_POINT('',(-0.008,-0.009,9.79717439317883E-19));
#31574=CARTESIAN_POINT('Origin',(0.,-0.00075000000001,0.));
#31575=CARTESIAN_POINT('Origin',(0.0155,-0.0607953551706409,0.0155));
#31576=CARTESIAN_POINT('',(0.0142705,-0.0607953551706409,0.0155));
#31577=CARTESIAN_POINT('Origin',(-0.0155,-0.0607953551706409,-0.0155));
#31578=CARTESIAN_POINT('',(-0.0167295,-0.0607953551706409,-0.0155));
#31579=CARTESIAN_POINT('Origin',(0.0155,-0.0607953551706409,-0.0155));
#31580=CARTESIAN_POINT('',(0.0142705,-0.0607953551706409,-0.0155));
#31581=CARTESIAN_POINT('Origin',(-0.0155,-0.0607953551706409,0.0155));
#31582=CARTESIAN_POINT('',(-0.0167295,-0.0607953551706409,0.0155));
#31583=CARTESIAN_POINT('Origin',(0.,-0.00075,0.));
#31584=CARTESIAN_POINT('',(-0.006,-0.00075000000001,7.34788079488412E-19));
#31585=CARTESIAN_POINT('Origin',(0.,-0.00075000000001,0.));
#31586=CARTESIAN_POINT('',(-0.006,-0.00075,7.34788079488412E-19));
#31587=CARTESIAN_POINT('Origin',(0.,-0.00075,0.));
#31588=CARTESIAN_POINT('Origin',(-0.0195,-0.008,-0.00807716446627536));
#31589=CARTESIAN_POINT('',(-0.01950000000001,-0.00800000000001,-0.00807716446628536));
#31590=CARTESIAN_POINT('Origin',(-0.00807716446627536,-0.008,-0.0195));
#31591=CARTESIAN_POINT('',(-0.00807716446628536,-0.00800000000001,-0.01950000000001));
#31592=CARTESIAN_POINT('Origin',(0.00807716446627536,-0.008,-0.0195));
#31593=CARTESIAN_POINT('',(0.00807716446628536,-0.00800000000001,-0.01950000000001));
#31594=CARTESIAN_POINT('Origin',(0.0195,-0.008,-0.00807716446627536));
#31595=CARTESIAN_POINT('Origin',(0.021,0.,0.016));
#34819=UNCERTAINTY_MEASURE_WITH_UNIT(LENGTH_MEASURE(1.E-5),#34877,
'DISTANCE_ACCURACY_VALUE',
'Maximum model space distance between geometric entities at asserted c
onnectivities');
#34841=UNCERTAINTY_MEASURE_WITH_UNIT(LENGTH_MEASURE(1.E-5),#34877,
'DISTANCE_ACCURACY_VALUE',
'Maximum model space distance between geometric entities at asserted c
onnectivities');
#34854=(
GEOMETRIC_REPRESENTATION_CONTEXT(3)
GLOBAL_UNCERTAINTY_ASSIGNED_CONTEXT((#34819))
GLOBAL_UNIT_ASSIGNED_CONTEXT((#34877,#34878,#34879))
REPRESENTATION_CONTEXT('','3D')
);
#34876=(
GEOMETRIC_REPRESENTATION_CONTEXT(3)
GLOBAL_UNCERTAINTY_ASSIGNED_CONTEXT((#34841))
GLOBAL_UNIT_ASSIGNED_CONTEXT((#34877,#34878,#34879))
REPRESENTATION_CONTEXT('','3D')
);
#34877=(
LENGTH_UNIT()
NAMED_UNIT(*)
SI_UNIT($,.METRE.)
);
#34878=(
NAMED_UNIT(*)
PLANE_ANGLE_UNIT()
SI_UNIT($,.RADIAN.)
);
#34879=(
NAMED_UNIT(*)
SI_UNIT($,.STERADIAN.)
SOLID_ANGLE_UNIT()
);
#34892=SHAPE_DEFINITION_REPRESENTATION(#34926,#34996);
#34926=PRODUCT_DEFINITION_SHAPE('',$,#35031);
#34996=SHAPE_REPRESENTATION('',(#20965),#34854);
#35018=PRODUCT_DEFINITION_CONTEXT('part definition',#35122,'design');
#35031=PRODUCT_DEFINITION('Motor Top Cap','Motor Top Cap',#35065,#35018);
#35065=PRODUCT_DEFINITION_FORMATION('',$,#35136);
#35122=APPLICATION_CONTEXT('Managed model based 3d engineering');
#35123=PRODUCT_CONTEXT('part definition',#35122,'mechanical');
#35136=PRODUCT('Motor Top Cap','Motor Top Cap',
'LEGAL AND USAGE DISCLAIMER: this Data/Model is provided \X2\201C\X0\A
S IS\X2\201D\X0\ for informational and representational only. It is a 
geometric approximation and is NOT engineered, certified, or guarantee
d for dimensional accuracy, exact tolerances, or production-level prec
ision. Vendor disclaims all implied warranties including fitness for a
 particular purpose. DO NOT USE FOR DIRECT PHYSICAL MANUFACTURING, AUT
OMATED PRODUCTION, OR SAFETY-CRITICAL SYSTEMS without independent engi
neering verification and resolution of any design discrepancies.',(#35123));
#35162=PRESENTATION_STYLE_ASSIGNMENT((#35171));
#35171=SURFACE_STYLE_USAGE(.BOTH.,#35180);
#35180=SURFACE_SIDE_STYLE('',(#35189));
#35189=SURFACE_STYLE_FILL_AREA(#35198);
#35198=FILL_AREA_STYLE('Aluminum - Anodized Glossy (Grey)',(#35207));
#35207=FILL_AREA_STYLE_COLOUR('Aluminum - Anodized Glossy (Grey)',#35216);
#35216=COLOUR_RGB('Aluminum - Anodized Glossy (Grey)',0.537254901960784,
0.537254901960784,0.537254901960784);
ENDSEC;
END-ISO-10303-21;
